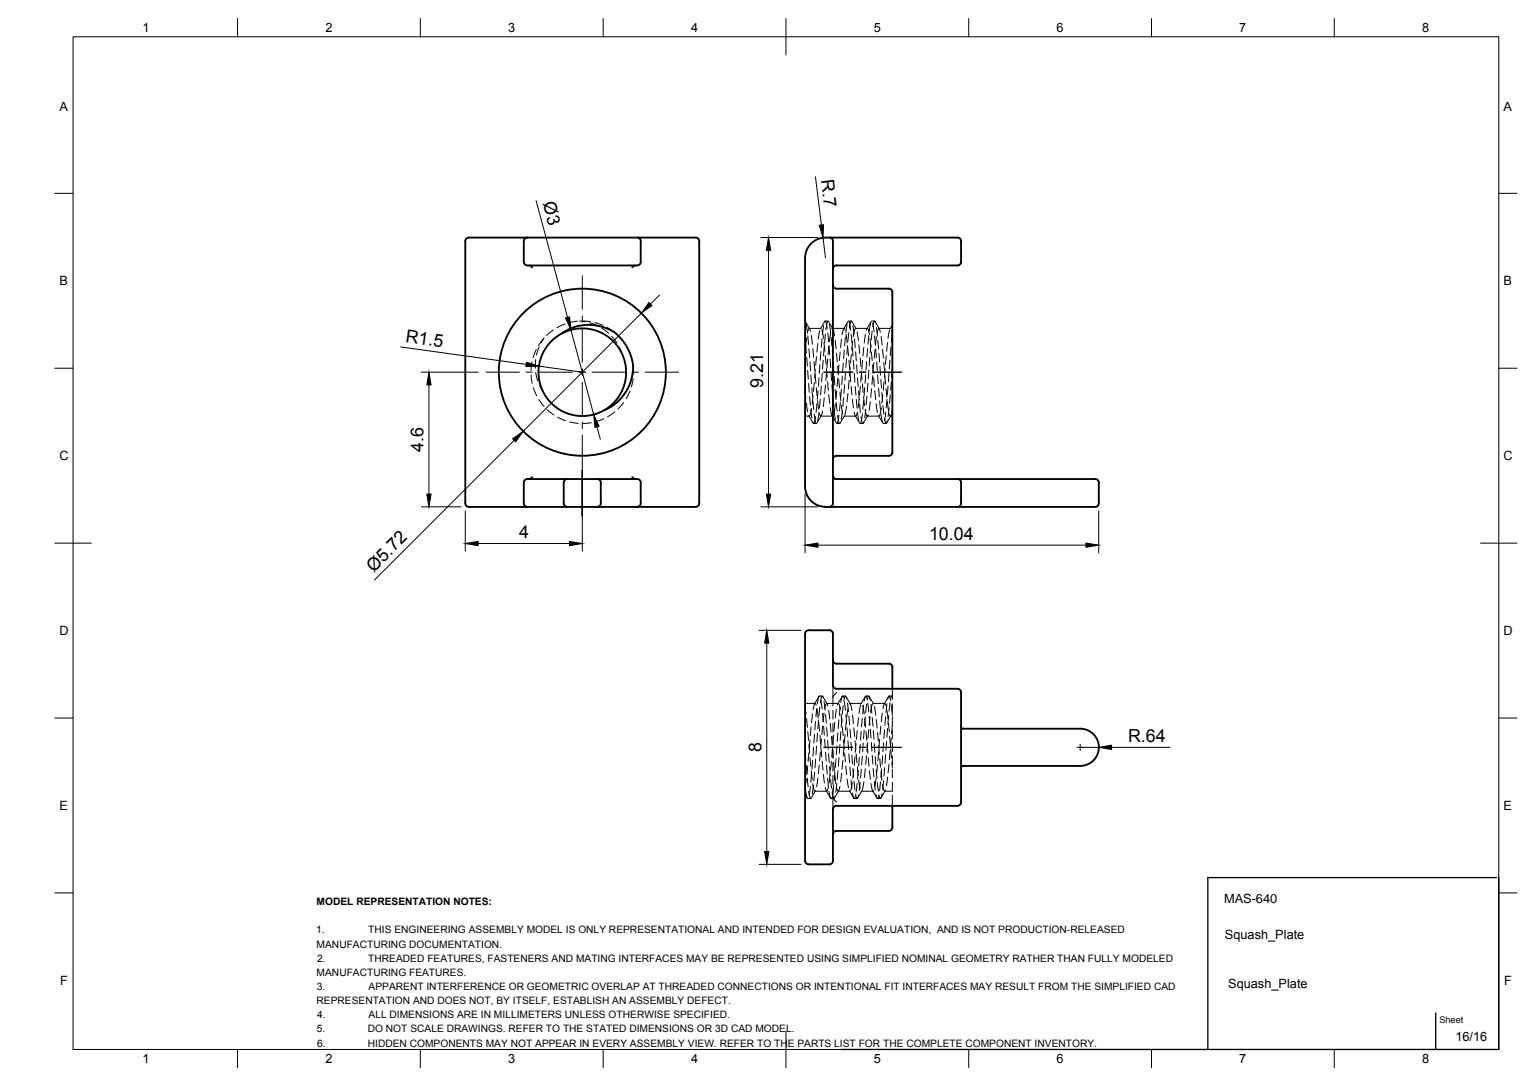
ISO-10303-21;
HEADER;
FILE_DESCRIPTION((''),'2;1');
FILE_NAME('Squash_Plate.step','2026-10-09T10:33:02-07:00',(''),(''),'','','');
FILE_SCHEMA (('AUTOMOTIVE_DESIGN { 1 0 10303 214 3 1 1 }'));
ENDSEC;
DATA;
#10=MECHANICAL_DESIGN_GEOMETRIC_PRESENTATION_REPRESENTATION('',(#844),#86330);
#109=SPHERICAL_SURFACE('',#35974,0.125) ;
#110=SPHERICAL_SURFACE('',#35976,0.125) ;
#111=SPHERICAL_SURFACE('',#35981,0.125) ;
#112=SPHERICAL_SURFACE('',#35983,0.125) ;
#113=SPHERICAL_SURFACE('',#36041,0.125) ;
#114=SPHERICAL_SURFACE('',#36047,0.125) ;
#115=SPHERICAL_SURFACE('',#36104,0.124999999999993) ;
#116=SPHERICAL_SURFACE('',#36105,0.125000000000011) ;
#117=SPHERICAL_SURFACE('',#36116,0.124999999999993) ;
#118=SPHERICAL_SURFACE('',#36117,0.124999999999993) ;
#119=SPHERICAL_SURFACE('',#36118,0.124999999999993) ;
#120=SPHERICAL_SURFACE('',#36119,0.124999999999993) ;
#436=TOROIDAL_SURFACE('',#35930,0.188499999999969,0.124999999999993) ;
#437=TOROIDAL_SURFACE('',#35937,0.188499999999987,0.124999999999993) ;
#438=TOROIDAL_SURFACE('',#35942,0.188499999999987,0.124999999999993) ;
#439=TOROIDAL_SURFACE('',#35949,0.509999999999996,0.125) ;
#440=TOROIDAL_SURFACE('',#35956,0.188499999999987,0.124999999999993) ;
#441=TOROIDAL_SURFACE('',#35965,0.509999999999996,0.125) ;
#442=TOROIDAL_SURFACE('',#36032,0.25,0.125) ;
#443=TOROIDAL_SURFACE('',#36035,0.25,0.125) ;
#444=TOROIDAL_SURFACE('',#36038,0.25,0.125) ;
#445=TOROIDAL_SURFACE('',#36044,0.25,0.125) ;
#446=TOROIDAL_SURFACE('',#36064,0.573499999999999,0.125) ;
#447=TOROIDAL_SURFACE('',#36068,0.573500000000001,0.125) ;
#448=TOROIDAL_SURFACE('',#36081,0.573500000000001,0.125) ;
#449=TOROIDAL_SURFACE('',#36085,0.573499999999999,0.125) ;
#450=TOROIDAL_SURFACE('',#36111,0.249999999999986,0.124999999999993) ;
#451=TOROIDAL_SURFACE('',#36115,0.250000000000004,0.124999999999993) ;
#452=TOROIDAL_SURFACE('',#36120,0.249999999999968,0.124999999999993) ;
#453=TOROIDAL_SURFACE('',#36121,0.249999999999986,0.124999999999993) ;
#454=TOROIDAL_SURFACE('',#36122,2.7325,0.125) ;
#455=TOROIDAL_SURFACE('',#36131,2.9825,0.125) ;
#746=(
BOUNDED_SURFACE()
B_SPLINE_SURFACE(1,2,((#79923,#79924,#79925,#79926,#79927,#79928,#79929,
#79930,#79931,#79932,#79933,#79934,#79935,#79936,#79937,#79938,#79939,#79940,
#79941,#79942,#79943,#79944,#79945,#79946,#79947,#79948,#79949,#79950,#79951,
#79952,#79953,#79954,#79955,#79956,#79957,#79958,#79959,#79960,#79961,#79962,
#79963,#79964,#79965,#79966,#79967,#79968,#79969,#79970,#79971,#79972,#79973,
#79974,#79975,#79976,#79977,#79978,#79979,#79980,#79981,#79982,#79983,#79984,
#79985,#79986,#79987,#79988,#79989,#79990,#79991,#79992,#79993,#79994,#79995,
#79996,#79997,#79998,#79999,#80000,#80001,#80002,#80003,#80004,#80005,#80006,
#80007,#80008,#80009,#80010,#80011,#80012,#80013,#80014,#80015,#80016,#80017,
#80018,#80019,#80020,#80021,#80022,#80023,#80024,#80025,#80026,#80027,#80028,
#80029,#80030,#80031,#80032,#80033,#80034,#80035,#80036,#80037,#80038,#80039,
#80040,#80041,#80042,#80043,#80044,#80045,#80046,#80047,#80048,#80049,#80050,
#80051,#80052,#80053,#80054,#80055,#80056,#80057,#80058,#80059,#80060,#80061,
#80062,#80063,#80064,#80065,#80066,#80067),(#80068,#80069,#80070,#80071,
#80072,#80073,#80074,#80075,#80076,#80077,#80078,#80079,#80080,#80081,#80082,
#80083,#80084,#80085,#80086,#80087,#80088,#80089,#80090,#80091,#80092,#80093,
#80094,#80095,#80096,#80097,#80098,#80099,#80100,#80101,#80102,#80103,#80104,
#80105,#80106,#80107,#80108,#80109,#80110,#80111,#80112,#80113,#80114,#80115,
#80116,#80117,#80118,#80119,#80120,#80121,#80122,#80123,#80124,#80125,#80126,
#80127,#80128,#80129,#80130,#80131,#80132,#80133,#80134,#80135,#80136,#80137,
#80138,#80139,#80140,#80141,#80142,#80143,#80144,#80145,#80146,#80147,#80148,
#80149,#80150,#80151,#80152,#80153,#80154,#80155,#80156,#80157,#80158,#80159,
#80160,#80161,#80162,#80163,#80164,#80165,#80166,#80167,#80168,#80169,#80170,
#80171,#80172,#80173,#80174,#80175,#80176,#80177,#80178,#80179,#80180,#80181,
#80182,#80183,#80184,#80185,#80186,#80187,#80188,#80189,#80190,#80191,#80192,
#80193,#80194,#80195,#80196,#80197,#80198,#80199,#80200,#80201,#80202,#80203,
#80204,#80205,#80206,#80207,#80208,#80209,#80210,#80211,#80212),(#80213,
#80214,#80215,#80216,#80217,#80218,#80219,#80220,#80221,#80222,#80223,#80224,
#80225,#80226,#80227,#80228,#80229,#80230,#80231,#80232,#80233,#80234,#80235,
#80236,#80237,#80238,#80239,#80240,#80241,#80242,#80243,#80244,#80245,#80246,
#80247,#80248,#80249,#80250,#80251,#80252,#80253,#80254,#80255,#80256,#80257,
#80258,#80259,#80260,#80261,#80262,#80263,#80264,#80265,#80266,#80267,#80268,
#80269,#80270,#80271,#80272,#80273,#80274,#80275,#80276,#80277,#80278,#80279,
#80280,#80281,#80282,#80283,#80284,#80285,#80286,#80287,#80288,#80289,#80290,
#80291,#80292,#80293,#80294,#80295,#80296,#80297,#80298,#80299,#80300,#80301,
#80302,#80303,#80304,#80305,#80306,#80307,#80308,#80309,#80310,#80311,#80312,
#80313,#80314,#80315,#80316,#80317,#80318,#80319,#80320,#80321,#80322,#80323,
#80324,#80325,#80326,#80327,#80328,#80329,#80330,#80331,#80332,#80333,#80334,
#80335,#80336,#80337,#80338,#80339,#80340,#80341,#80342,#80343,#80344,#80345,
#80346,#80347,#80348,#80349,#80350,#80351,#80352,#80353,#80354,#80355,#80356,
#80357),(#80358,#80359,#80360,#80361,#80362,#80363,#80364,#80365,#80366,
#80367,#80368,#80369,#80370,#80371,#80372,#80373,#80374,#80375,#80376,#80377,
#80378,#80379,#80380,#80381,#80382,#80383,#80384,#80385,#80386,#80387,#80388,
#80389,#80390,#80391,#80392,#80393,#80394,#80395,#80396,#80397,#80398,#80399,
#80400,#80401,#80402,#80403,#80404,#80405,#80406,#80407,#80408,#80409,#80410,
#80411,#80412,#80413,#80414,#80415,#80416,#80417,#80418,#80419,#80420,#80421,
#80422,#80423,#80424,#80425,#80426,#80427,#80428,#80429,#80430,#80431,#80432,
#80433,#80434,#80435,#80436,#80437,#80438,#80439,#80440,#80441,#80442,#80443,
#80444,#80445,#80446,#80447,#80448,#80449,#80450,#80451,#80452,#80453,#80454,
#80455,#80456,#80457,#80458,#80459,#80460,#80461,#80462,#80463,#80464,#80465,
#80466,#80467,#80468,#80469,#80470,#80471,#80472,#80473,#80474,#80475,#80476,
#80477,#80478,#80479,#80480,#80481,#80482,#80483,#80484,#80485,#80486,#80487,
#80488,#80489,#80490,#80491,#80492,#80493,#80494,#80495,#80496,#80497,#80498,
#80499,#80500,#80501,#80502)),.UNSPECIFIED.,.F.,.F.,.F.)
B_SPLINE_SURFACE_WITH_KNOTS((2,1,1,2),(3,2,2,2,2,2,2,2,2,2,2,2,2,2,2,2,
2,2,2,2,2,2,2,2,2,2,2,2,2,2,2,2,2,2,2,2,2,2,2,2,2,2,2,2,2,2,2,2,2,2,2,2,
2,2,2,2,2,2,2,2,2,2,2,2,2,2,2,2,2,2,2,2,3),(-5.32860868657006,0.,1.,2.58924025826637),
(0.,0.0138888888888889,0.0277777777777778,0.0416666666666667,0.0555555555555556,
0.0694444444444444,0.0833333333333333,0.0972222222222222,0.111111111111111,
0.125,0.138888888888889,0.152777777777778,0.166666666666667,0.180555555555556,
0.194444444444444,0.208333333333333,0.222222222222222,0.236111111111111,
0.25,0.263888888888889,0.277777777777778,0.291666666666667,0.305555555555556,
0.319444444444444,0.333333333333333,0.347222222222222,0.361111111111111,
0.375,0.388888888888889,0.402777777777778,0.416666666666667,0.430555555555556,
0.444444444444444,0.458333333333333,0.472222222222222,0.486111111111111,
0.5,0.513888888888889,0.527777777777778,0.541666666666667,0.555555555555556,
0.569444444444444,0.583333333333333,0.597222222222222,0.611111111111111,
0.625,0.638888888888889,0.652777777777778,0.666666666666667,0.680555555555556,
0.694444444444444,0.708333333333333,0.722222222222222,0.736111111111111,
0.75,0.763888888888889,0.777777777777778,0.791666666666667,0.805555555555556,
0.819444444444444,0.833333333333333,0.847222222222222,0.861111111111111,
0.875,0.888888888888889,0.902777777777778,0.916666666666667,0.930555555555556,
0.944444444444444,0.958333333333333,0.972222222222222,0.986111111111111,
1.),.UNSPECIFIED.)
GEOMETRIC_REPRESENTATION_ITEM()
RATIONAL_B_SPLINE_SURFACE(((1.,0.923879532511287,1.,0.923879532511287,1.,
0.923879532511287,1.,0.923879532511287,1.,0.923879532511287,1.,0.923879532511287,
1.,0.923879532511287,1.,0.923879532511287,1.,0.923879532511287,1.,0.923879532511287,
1.,0.923879532511287,1.,0.923879532511287,1.,0.923879532511287,1.,0.923879532511287,
1.,0.923879532511287,1.,0.923879532511287,1.,0.923879532511287,1.,0.923879532511287,
1.,0.923879532511287,1.,0.923879532511287,1.,0.923879532511287,1.,0.923879532511287,
1.,0.923879532511287,1.,0.923879532511287,1.,0.923879532511287,1.,0.923879532511287,
1.,0.923879532511287,1.,0.923879532511287,1.,0.923879532511287,1.,0.923879532511287,
1.,0.923879532511287,1.,0.923879532511287,1.,0.923879532511287,1.,0.923879532511287,
1.,0.923879532511287,1.,0.923879532511287,1.,0.923879532511287,1.,0.923879532511287,
1.,0.923879532511287,1.,0.923879532511287,1.,0.923879532511287,1.,0.923879532511287,
1.,0.923879532511287,1.,0.923879532511287,1.,0.923879532511287,1.,0.923879532511287,
1.,0.923879532511287,1.,0.923879532511287,1.,0.923879532511287,1.,0.923879532511287,
1.,0.923879532511287,1.,0.923879532511287,1.,0.923879532511287,1.,0.923879532511287,
1.,0.923879532511287,1.,0.923879532511287,1.,0.923879532511287,1.,0.923879532511287,
1.,0.923879532511287,1.,0.923879532511287,1.,0.923879532511287,1.,0.923879532511287,
1.,0.923879532511287,1.,0.923879532511287,1.,0.923879532511287,1.,0.923879532511287,
1.,0.923879532511287,1.,0.923879532511287,1.,0.923879532511287,1.,0.923879532511287,
1.,0.923879532511287,1.,0.923879532511287,1.),(1.,0.923879532511287,1.,
0.923879532511287,1.,0.923879532511287,1.,0.923879532511287,1.,0.923879532511287,
1.,0.923879532511287,1.,0.923879532511287,1.,0.923879532511287,1.,0.923879532511287,
1.,0.923879532511287,1.,0.923879532511287,1.,0.923879532511287,1.,0.923879532511287,
1.,0.923879532511287,1.,0.923879532511287,1.,0.923879532511287,1.,0.923879532511287,
1.,0.923879532511287,1.,0.923879532511287,1.,0.923879532511287,1.,0.923879532511287,
1.,0.923879532511287,1.,0.923879532511287,1.,0.923879532511287,1.,0.923879532511287,
1.,0.923879532511287,1.,0.923879532511287,1.,0.923879532511287,1.,0.923879532511287,
1.,0.923879532511287,1.,0.923879532511287,1.,0.923879532511287,1.,0.923879532511287,
1.,0.923879532511287,1.,0.923879532511287,1.,0.923879532511287,1.,0.923879532511287,
1.,0.923879532511287,1.,0.923879532511287,1.,0.923879532511287,1.,0.923879532511287,
1.,0.923879532511287,1.,0.923879532511287,1.,0.923879532511287,1.,0.923879532511287,
1.,0.923879532511287,1.,0.923879532511287,1.,0.923879532511287,1.,0.923879532511287,
1.,0.923879532511287,1.,0.923879532511287,1.,0.923879532511287,1.,0.923879532511287,
1.,0.923879532511287,1.,0.923879532511287,1.,0.923879532511287,1.,0.923879532511287,
1.,0.923879532511287,1.,0.923879532511287,1.,0.923879532511287,1.,0.923879532511287,
1.,0.923879532511287,1.,0.923879532511287,1.,0.923879532511287,1.,0.923879532511287,
1.,0.923879532511287,1.,0.923879532511287,1.,0.923879532511287,1.,0.923879532511287,
1.,0.923879532511287,1.,0.923879532511287,1.,0.923879532511287,1.),(1.,
0.923879532511287,1.,0.923879532511287,1.,0.923879532511287,1.,0.923879532511287,
1.,0.923879532511287,1.,0.923879532511287,1.,0.923879532511287,1.,0.923879532511287,
1.,0.923879532511287,1.,0.923879532511287,1.,0.923879532511287,1.,0.923879532511287,
1.,0.923879532511287,1.,0.923879532511287,1.,0.923879532511287,1.,0.923879532511287,
1.,0.923879532511287,1.,0.923879532511287,1.,0.923879532511287,1.,0.923879532511287,
1.,0.923879532511287,1.,0.923879532511287,1.,0.923879532511287,1.,0.923879532511287,
1.,0.923879532511287,1.,0.923879532511287,1.,0.923879532511287,1.,0.923879532511287,
1.,0.923879532511287,1.,0.923879532511287,1.,0.923879532511287,1.,0.923879532511287,
1.,0.923879532511287,1.,0.923879532511287,1.,0.923879532511287,1.,0.923879532511287,
1.,0.923879532511287,1.,0.923879532511287,1.,0.923879532511287,1.,0.923879532511287,
1.,0.923879532511287,1.,0.923879532511287,1.,0.923879532511287,1.,0.923879532511287,
1.,0.923879532511287,1.,0.923879532511287,1.,0.923879532511287,1.,0.923879532511287,
1.,0.923879532511287,1.,0.923879532511287,1.,0.923879532511287,1.,0.923879532511287,
1.,0.923879532511287,1.,0.923879532511287,1.,0.923879532511287,1.,0.923879532511287,
1.,0.923879532511287,1.,0.923879532511287,1.,0.923879532511287,1.,0.923879532511287,
1.,0.923879532511287,1.,0.923879532511287,1.,0.923879532511287,1.,0.923879532511287,
1.,0.923879532511287,1.,0.923879532511287,1.,0.923879532511287,1.,0.923879532511287,
1.,0.923879532511287,1.,0.923879532511287,1.,0.923879532511287,1.,0.923879532511287,
1.),(1.,0.923879532511287,1.,0.923879532511287,1.,0.923879532511287,1.,
0.923879532511287,1.,0.923879532511287,1.,0.923879532511287,1.,0.923879532511287,
1.,0.923879532511287,1.,0.923879532511287,1.,0.923879532511287,1.,0.923879532511287,
1.,0.923879532511287,1.,0.923879532511287,1.,0.923879532511287,1.,0.923879532511287,
1.,0.923879532511287,1.,0.923879532511287,1.,0.923879532511287,1.,0.923879532511287,
1.,0.923879532511287,1.,0.923879532511287,1.,0.923879532511287,1.,0.923879532511287,
1.,0.923879532511287,1.,0.923879532511287,1.,0.923879532511287,1.,0.923879532511287,
1.,0.923879532511287,1.,0.923879532511287,1.,0.923879532511287,1.,0.923879532511287,
1.,0.923879532511287,1.,0.923879532511287,1.,0.923879532511287,1.,0.923879532511287,
1.,0.923879532511287,1.,0.923879532511287,1.,0.923879532511287,1.,0.923879532511287,
1.,0.923879532511287,1.,0.923879532511287,1.,0.923879532511287,1.,0.923879532511287,
1.,0.923879532511287,1.,0.923879532511287,1.,0.923879532511287,1.,0.923879532511287,
1.,0.923879532511287,1.,0.923879532511287,1.,0.923879532511287,1.,0.923879532511287,
1.,0.923879532511287,1.,0.923879532511287,1.,0.923879532511287,1.,0.923879532511287,
1.,0.923879532511287,1.,0.923879532511287,1.,0.923879532511287,1.,0.923879532511287,
1.,0.923879532511287,1.,0.923879532511287,1.,0.923879532511287,1.,0.923879532511287,
1.,0.923879532511287,1.,0.923879532511287,1.,0.923879532511287,1.,0.923879532511287,
1.,0.923879532511287,1.,0.923879532511287,1.,0.923879532511287,1.,0.923879532511287,
1.,0.923879532511287,1.)))
REPRESENTATION_ITEM('')
SURFACE()
) ;
#747=(
BOUNDED_SURFACE()
B_SPLINE_SURFACE(1,2,((#80503,#80504,#80505,#80506,#80507,#80508,#80509,
#80510,#80511,#80512,#80513,#80514,#80515,#80516,#80517,#80518,#80519,#80520,
#80521,#80522,#80523,#80524,#80525,#80526,#80527,#80528,#80529,#80530,#80531,
#80532,#80533,#80534,#80535,#80536,#80537,#80538,#80539,#80540,#80541,#80542,
#80543,#80544,#80545,#80546,#80547,#80548,#80549,#80550,#80551,#80552,#80553,
#80554,#80555,#80556,#80557,#80558,#80559,#80560,#80561,#80562,#80563,#80564,
#80565,#80566,#80567,#80568,#80569,#80570,#80571,#80572,#80573,#80574,#80575,
#80576,#80577,#80578,#80579,#80580,#80581,#80582,#80583,#80584,#80585,#80586,
#80587,#80588,#80589,#80590,#80591,#80592,#80593,#80594,#80595,#80596,#80597,
#80598,#80599,#80600,#80601,#80602,#80603,#80604,#80605,#80606,#80607,#80608,
#80609,#80610,#80611,#80612,#80613,#80614,#80615,#80616,#80617,#80618,#80619,
#80620,#80621,#80622,#80623,#80624,#80625,#80626,#80627,#80628,#80629,#80630,
#80631,#80632,#80633,#80634,#80635,#80636,#80637,#80638,#80639,#80640,#80641,
#80642,#80643,#80644,#80645,#80646,#80647),(#80648,#80649,#80650,#80651,
#80652,#80653,#80654,#80655,#80656,#80657,#80658,#80659,#80660,#80661,#80662,
#80663,#80664,#80665,#80666,#80667,#80668,#80669,#80670,#80671,#80672,#80673,
#80674,#80675,#80676,#80677,#80678,#80679,#80680,#80681,#80682,#80683,#80684,
#80685,#80686,#80687,#80688,#80689,#80690,#80691,#80692,#80693,#80694,#80695,
#80696,#80697,#80698,#80699,#80700,#80701,#80702,#80703,#80704,#80705,#80706,
#80707,#80708,#80709,#80710,#80711,#80712,#80713,#80714,#80715,#80716,#80717,
#80718,#80719,#80720,#80721,#80722,#80723,#80724,#80725,#80726,#80727,#80728,
#80729,#80730,#80731,#80732,#80733,#80734,#80735,#80736,#80737,#80738,#80739,
#80740,#80741,#80742,#80743,#80744,#80745,#80746,#80747,#80748,#80749,#80750,
#80751,#80752,#80753,#80754,#80755,#80756,#80757,#80758,#80759,#80760,#80761,
#80762,#80763,#80764,#80765,#80766,#80767,#80768,#80769,#80770,#80771,#80772,
#80773,#80774,#80775,#80776,#80777,#80778,#80779,#80780,#80781,#80782,#80783,
#80784,#80785,#80786,#80787,#80788,#80789,#80790,#80791,#80792)),
 .UNSPECIFIED.,.F.,.F.,.F.)
B_SPLINE_SURFACE_WITH_KNOTS((2,2),(3,2,2,2,2,2,2,2,2,2,2,2,2,2,2,2,2,2,
2,2,2,2,2,2,2,2,2,2,2,2,2,2,2,2,2,2,2,2,2,2,2,2,2,2,2,2,2,2,2,2,2,2,2,2,
2,2,2,2,2,2,2,2,2,2,2,2,2,2,2,2,2,2,3),(0.,1.00004424589271),(0.,0.0138888888888889,
0.0277777777777778,0.0416666666666667,0.0555555555555556,0.0694444444444444,
0.0833333333333333,0.0972222222222222,0.111111111111111,0.125,0.138888888888889,
0.152777777777778,0.166666666666667,0.180555555555556,0.194444444444444,
0.208333333333333,0.222222222222222,0.236111111111111,0.25,0.263888888888889,
0.277777777777778,0.291666666666667,0.305555555555556,0.319444444444444,
0.333333333333333,0.347222222222222,0.361111111111111,0.375,0.388888888888889,
0.402777777777778,0.416666666666667,0.430555555555556,0.444444444444444,
0.458333333333333,0.472222222222222,0.486111111111111,0.5,0.513888888888889,
0.527777777777778,0.541666666666667,0.555555555555556,0.569444444444444,
0.583333333333333,0.597222222222222,0.611111111111111,0.625,0.638888888888889,
0.652777777777778,0.666666666666667,0.680555555555556,0.694444444444444,
0.708333333333333,0.722222222222222,0.736111111111111,0.75,0.763888888888889,
0.777777777777778,0.791666666666667,0.805555555555556,0.819444444444444,
0.833333333333333,0.847222222222222,0.861111111111111,0.875,0.888888888888889,
0.902777777777778,0.916666666666667,0.930555555555556,0.944444444444444,
0.958333333333333,0.972222222222222,0.986111111111111,1.),.UNSPECIFIED.)
GEOMETRIC_REPRESENTATION_ITEM()
RATIONAL_B_SPLINE_SURFACE(((1.,0.923879532511287,1.,0.923879532511287,1.,
0.923879532511287,1.,0.923879532511287,1.,0.923879532511287,1.,0.923879532511287,
1.,0.923879532511287,1.,0.923879532511287,1.,0.923879532511287,1.,0.923879532511287,
1.,0.923879532511287,1.,0.923879532511287,1.,0.923879532511287,1.,0.923879532511287,
1.,0.923879532511287,1.,0.923879532511287,1.,0.923879532511287,1.,0.923879532511287,
1.,0.923879532511287,1.,0.923879532511287,1.,0.923879532511287,1.,0.923879532511287,
1.,0.923879532511287,1.,0.923879532511287,1.,0.923879532511287,1.,0.923879532511287,
1.,0.923879532511287,1.,0.923879532511287,1.,0.923879532511287,1.,0.923879532511287,
1.,0.923879532511287,1.,0.923879532511287,1.,0.923879532511287,1.,0.923879532511287,
1.,0.923879532511287,1.,0.923879532511287,1.,0.923879532511287,1.,0.923879532511287,
1.,0.923879532511287,1.,0.923879532511287,1.,0.923879532511287,1.,0.923879532511287,
1.,0.923879532511287,1.,0.923879532511287,1.,0.923879532511287,1.,0.923879532511287,
1.,0.923879532511287,1.,0.923879532511287,1.,0.923879532511287,1.,0.923879532511287,
1.,0.923879532511287,1.,0.923879532511287,1.,0.923879532511287,1.,0.923879532511287,
1.,0.923879532511287,1.,0.923879532511287,1.,0.923879532511287,1.,0.923879532511287,
1.,0.923879532511287,1.,0.923879532511287,1.,0.923879532511287,1.,0.923879532511287,
1.,0.923879532511287,1.,0.923879532511287,1.,0.923879532511287,1.,0.923879532511287,
1.,0.923879532511287,1.,0.923879532511287,1.,0.923879532511287,1.,0.923879532511287,
1.,0.923879532511287,1.,0.923879532511287,1.),(1.,0.923879532511287,1.,
0.923879532511287,1.,0.923879532511287,1.,0.923879532511287,1.,0.923879532511287,
1.,0.923879532511287,1.,0.923879532511287,1.,0.923879532511287,1.,0.923879532511287,
1.,0.923879532511287,1.,0.923879532511287,1.,0.923879532511287,1.,0.923879532511287,
1.,0.923879532511287,1.,0.923879532511287,1.,0.923879532511287,1.,0.923879532511287,
1.,0.923879532511287,1.,0.923879532511287,1.,0.923879532511287,1.,0.923879532511287,
1.,0.923879532511287,1.,0.923879532511287,1.,0.923879532511287,1.,0.923879532511287,
1.,0.923879532511287,1.,0.923879532511287,1.,0.923879532511287,1.,0.923879532511287,
1.,0.923879532511287,1.,0.923879532511287,1.,0.923879532511287,1.,0.923879532511287,
1.,0.923879532511287,1.,0.923879532511287,1.,0.923879532511287,1.,0.923879532511287,
1.,0.923879532511287,1.,0.923879532511287,1.,0.923879532511287,1.,0.923879532511287,
1.,0.923879532511287,1.,0.923879532511287,1.,0.923879532511287,1.,0.923879532511287,
1.,0.923879532511287,1.,0.923879532511287,1.,0.923879532511287,1.,0.923879532511287,
1.,0.923879532511287,1.,0.923879532511287,1.,0.923879532511287,1.,0.923879532511287,
1.,0.923879532511287,1.,0.923879532511287,1.,0.923879532511287,1.,0.923879532511287,
1.,0.923879532511287,1.,0.923879532511287,1.,0.923879532511287,1.,0.923879532511287,
1.,0.923879532511287,1.,0.923879532511287,1.,0.923879532511287,1.,0.923879532511287,
1.,0.923879532511287,1.,0.923879532511287,1.,0.923879532511287,1.,0.923879532511287,
1.,0.923879532511287,1.,0.923879532511287,1.,0.923879532511287,1.)))
REPRESENTATION_ITEM('')
SURFACE()
) ;
#820=SHAPE_REPRESENTATION_RELATIONSHIP('SRR','None',#86465,#832) ;
#832=ADVANCED_BREP_SHAPE_REPRESENTATION('',(#856),#86319) ;
#844=STYLED_ITEM('',(#86582),#856) ;
#856=MANIFOLD_SOLID_BREP('Body1',#32643) ;
#1170=FACE_BOUND('',#5960,.T.) ;
#1171=FACE_BOUND('',#6015,.T.) ;
#1172=FACE_BOUND('',#6019,.T.) ;
#1580=B_SPLINE_CURVE_WITH_KNOTS('',3,(#78793,#78794,#78795,#78796,#78797,
#78798,#78799,#78800,#78801,#78802,#78803,#78804,#78805,#78806,#78807,#78808),
 .UNSPECIFIED.,.F.,.F.,(4,2,2,2,2,2,2,4),(3.73678905355268,3.77583604564174,
3.84429316886454,3.9117839455625,3.98028517515954,4.04771812918815,4.09356285357691,
4.13893020482044),.UNSPECIFIED.) ;
#1581=B_SPLINE_CURVE_WITH_KNOTS('',3,(#78811,#78812,#78813,#78814,#78815,
#78816,#78817,#78818,#78819,#78820,#78821,#78822,#78823,#78824,#78825,#78826,
#78827,#78828,#78829,#78830),.UNSPECIFIED.,.F.,.F.,(4,2,2,2,2,2,2,2,2,4),
(1.00000010744283E-6,0.0499431784479235,0.100287210935025,0.168054642610065,
0.237494946806667,0.305292985567466,0.374683046548786,0.442516172111994,
0.51185655028286,0.544247303702404),.UNSPECIFIED.) ;
#1582=B_SPLINE_CURVE_WITH_KNOTS('',3,(#78835,#78836,#78837,#78838,#78839,
#78840,#78841,#78842,#78843,#78844,#78845,#78846,#78847,#78848,#78849,#78850,
#78851,#78852,#78853,#78854,#78855,#78856,#78857,#78858,#78859,#78860,#78861,
#78862,#78863,#78864,#78865,#78866,#78867,#78868,#78869,#78870),
 .UNSPECIFIED.,.F.,.F.,(4,2,2,2,2,2,2,2,2,2,2,2,2,2,2,2,2,4),(2.63879249403916,
2.68716207519284,2.75533111613759,2.82339735412774,2.89159459627009,2.95958001185233,
3.02780800755272,3.09571469311715,3.1639758471015,3.23180612291199,3.30010268233795,
3.36785909776552,3.43619314464488,3.50387847678256,3.57225192300491,3.63986917252862,
3.70828375765117,3.73678905355268),.UNSPECIFIED.) ;
#1583=B_SPLINE_CURVE_WITH_KNOTS('',3,(#78871,#78872,#78873,#78874,#78875,
#78876,#78877,#78878,#78879,#78880,#78881,#78882,#78883,#78884,#78885,#78886,
#78887,#78888,#78889,#78890,#78891,#78892,#78893,#78894,#78895,#78896,#78897,
#78898,#78899,#78900,#78901,#78902,#78903,#78904,#78905,#78906),
 .UNSPECIFIED.,.F.,.F.,(4,2,2,2,2,2,2,2,2,2,2,2,2,2,2,2,2,4),(0.544247303702404,
0.579729241383105,0.649020714981666,0.71693728891309,0.786180492040209,
0.854145311540051,0.923341134445988,0.991358342360499,1.06050780118652,
1.12858131963186,1.19768557917167,1.26581915872125,1.33487954264344,1.40307674572091,
1.47209474432328,1.54035893111266,1.6093362063892,1.65177826841052),
 .UNSPECIFIED.) ;
#1584=B_SPLINE_CURVE_WITH_KNOTS('',3,(#78911,#78912,#78913,#78914,#78915,
#78916,#78917,#78918,#78919,#78920,#78921,#78922,#78923,#78924,#78925,#78926,
#78927,#78928,#78929,#78930,#78931,#78932,#78933,#78934,#78935,#78936,#78937,
#78938,#78939,#78940,#78941,#78942,#78943,#78944,#78945,#78946),
 .UNSPECIFIED.,.F.,.F.,(4,2,2,2,2,2,2,2,2,2,2,2,2,2,2,2,2,4),(1.5389994522091,
1.59333149801295,1.66297884651135,1.7301821776633,1.79977280875785,1.86694772145314,
1.93648225696496,2.00363195036966,2.07311098033212,2.14160511265088,2.20968937196864,
2.27809543856464,2.34619647664059,2.41451552535451,2.48263634985671,2.55086961886095,
2.61901314661333,2.63879249403916),.UNSPECIFIED.) ;
#1585=B_SPLINE_CURVE_WITH_KNOTS('',3,(#78947,#78948,#78949,#78950,#78951,
#78952,#78953,#78954,#78955,#78956,#78957,#78958,#78959,#78960,#78961,#78962,
#78963,#78964,#78965,#78966,#78967,#78968,#78969,#78970,#78971,#78972,#78973,
#78974,#78975,#78976,#78977,#78978,#78979,#78980,#78981,#78982),
 .UNSPECIFIED.,.F.,.F.,(4,2,2,2,2,2,2,2,2,2,2,2,2,2,2,2,2,4),(1.65177826841052,
1.6776705234471,1.7466089112996,1.81501628298846,1.8839177925435,1.95240091532547,
2.02126772540027,2.08982906495714,2.15959253692843,2.22727314697463,2.29708965878139,
2.36477169799653,2.43464163209697,2.50232925343889,2.57225301932284,2.63995025192664,
2.70992829083685,2.76015985424245),.UNSPECIFIED.) ;
#1586=B_SPLINE_CURVE_WITH_KNOTS('',3,(#78988,#78989,#78990,#78991,#78992,
#78993,#78994,#78995,#78996,#78997,#78998,#78999,#79000,#79001),
 .UNSPECIFIED.,.F.,.F.,(4,2,2,2,2,2,4),(3.87088446641146,3.88207110309913,
3.95256288258768,4.02054495054698,4.09109719843181,4.13081697342442,4.16975042780213),
 .UNSPECIFIED.) ;
#1587=B_SPLINE_CURVE_WITH_KNOTS('',3,(#79004,#79005,#79006,#79007,#79008,
#79009,#79010,#79011,#79012,#79013,#79014,#79015,#79016,#79017,#79018,#79019,
#79020,#79021),.UNSPECIFIED.,.F.,.F.,(4,2,2,2,2,2,2,2,4),(9.99925951688718E-7,
0.0402770593329322,0.0813965593939245,0.151714020497245,0.219397414529146,
0.289650306659335,0.357279908909674,0.427468950574574,0.435597230048873),
 .UNSPECIFIED.) ;
#1588=B_SPLINE_CURVE_WITH_KNOTS('',3,(#79027,#79028,#79029,#79030,#79031,
#79032,#79033,#79034,#79035,#79036),.UNSPECIFIED.,.F.,.F.,(4,2,2,2,4),(-0.1667127750087,
-0.142097710392982,-0.0825624075964315,-0.0415013685793908,-1.00000012634438E-6),
 .UNSPECIFIED.) ;
#1589=B_SPLINE_CURVE_WITH_KNOTS('',3,(#79039,#79040,#79041,#79042,#79043,
#79044,#79045,#79046,#79047,#79048,#79049,#79050,#79051,#79052,#79053,#79054,
#79055,#79056,#79057,#79058,#79059,#79060,#79061,#79062,#79063,#79064),
 .UNSPECIFIED.,.F.,.F.,(4,2,2,2,2,2,2,2,2,2,2,2,4),(-3.52511524228821,-3.4879111620666,
-3.45147286206197,-3.39356408207001,-3.33588355377615,-3.27799407259938,
-3.22024929076642,-3.16237686440599,-3.10456617477217,-3.04670845322558,
-2.98883032321556,-2.9309848603785,-2.88876551162052),.UNSPECIFIED.) ;
#1590=B_SPLINE_CURVE_WITH_KNOTS('',3,(#79069,#79070,#79071,#79072,#79073,
#79074,#79075,#79076,#79077,#79078,#79079,#79080,#79081,#79082,#79083,#79084,
#79085,#79086,#79087,#79088,#79089,#79090,#79091,#79092,#79093,#79094,#79095,
#79096,#79097,#79098,#79099,#79100,#79101,#79102,#79103,#79104),
 .UNSPECIFIED.,.F.,.F.,(4,2,2,2,2,2,2,2,2,2,2,2,2,2,2,2,2,4),(-1.1147036297923,
-1.08234127378787,-1.0231056786126,-0.964814237103067,-0.905544180711381,
-0.847294503532792,-0.787988947858243,-0.729777999922997,-0.670436005006492,
-0.612260463830717,-0.552881168011551,-0.494737717697047,-0.435320348351732,
-0.377205696945116,-0.317749544705521,-0.259660335123111,-0.200164740500403,
-0.1667127750087),.UNSPECIFIED.) ;
#1591=B_SPLINE_CURVE_WITH_KNOTS('',3,(#79105,#79106,#79107,#79108,#79109,
#79110,#79111,#79112,#79113,#79114,#79115,#79116,#79117,#79118,#79119,#79120,
#79121,#79122,#79123,#79124,#79125,#79126,#79127,#79128,#79129,#79130,#79131,
#79132,#79133,#79134,#79135,#79136,#79137,#79138,#79139,#79140),
 .UNSPECIFIED.,.F.,.F.,(4,2,2,2,2,2,2,2,2,2,2,2,2,2,2,2,2,4),(-2.88876551162052,
-2.8730378509001,-2.81520202632923,-2.75718479476445,-2.69935609300128,
-2.64126751092778,-2.58344326618254,-2.52528224276112,-2.46745974068091,
-2.40922528204208,-2.35140177232791,-2.2930929756667,-2.23526568453019,
-2.17688173210656,-2.1190478743858,-2.06058802751593,-2.00274481828321,
-1.95515401212426),.UNSPECIFIED.) ;
#1592=B_SPLINE_CURVE_WITH_KNOTS('',3,(#79145,#79146,#79147,#79148,#79149,
#79150,#79151,#79152,#79153,#79154,#79155,#79156,#79157,#79158,#79159,#79160,
#79161,#79162,#79163,#79164,#79165,#79166,#79167,#79168,#79169,#79170,#79171,
#79172,#79173,#79174,#79175,#79176,#79177,#79178,#79179,#79180),
 .UNSPECIFIED.,.F.,.F.,(4,2,2,2,2,2,2,2,2,2,2,2,2,2,2,2,2,4),(-2.06310075398818,
-2.02342933420803,-1.96363930695818,-1.90563613528142,-1.8458898927228,
-1.78788604802015,-1.72882872991433,-1.6702291728422,-1.61114617975511,
-1.5526042180681,-1.49349375729761,-1.43500706290225,-1.37586747600671,
-1.31743359143829,-1.25826335363796,-1.19987969503678,-1.1406774124604,
-1.1147036297923),.UNSPECIFIED.) ;
#1593=B_SPLINE_CURVE_WITH_KNOTS('',3,(#79181,#79182,#79183,#79184,#79185,
#79186,#79187,#79188,#79189,#79190,#79191,#79192,#79193,#79194,#79195,#79196,
#79197,#79198,#79199,#79200,#79201,#79202,#79203,#79204,#79205,#79206,#79207,
#79208,#79209,#79210,#79211,#79212,#79213,#79214,#79215,#79216),
 .UNSPECIFIED.,.F.,.F.,(4,2,2,2,2,2,2,2,2,2,2,2,2,2,2,2,2,4),(-1.95515401212426,
-1.94420841138501,-1.88635307691628,-1.82773951167999,-1.76986929968893,
-1.71260942538492,-1.65318316629389,-1.59587567208381,-1.53639019675408,
-1.47903330179993,-1.41948762790906,-1.36207963998264,-1.3024728018388,
-1.24501211437446,-1.18534316543117,-1.12782825442788,-1.06809626943629,
-1.01710396538768),.UNSPECIFIED.) ;
#1594=B_SPLINE_CURVE_WITH_KNOTS('',3,(#79222,#79223,#79224,#79225,#79226,
#79227,#79228,#79229),.UNSPECIFIED.,.F.,.F.,(4,2,2,4),(-0.0724080849059257,
-0.0675792623524678,-0.0340552227594196,-9.99999997836065E-7),
 .UNSPECIFIED.) ;
#1595=B_SPLINE_CURVE_WITH_KNOTS('',3,(#79232,#79233,#79234,#79235,#79236,
#79237,#79238,#79239,#79240,#79241,#79242,#79243,#79244,#79245,#79246,#79247,
#79248,#79249,#79250,#79251,#79252,#79253,#79254,#79255),.UNSPECIFIED.,
 .F.,.F.,(4,2,2,2,2,2,2,2,2,2,2,4),(-3.56932824666088,-3.53449866700443,
-3.50005253731909,-3.44177237096352,-3.38139391611913,-3.32315169324715,
-3.26282744772412,-3.2046207539918,-3.14434969751453,-3.08617601623974,
-3.02595714369959,-3.01323089524153),.UNSPECIFIED.) ;
#1596=B_SPLINE_CURVE_WITH_KNOTS('',3,(#79257,#79258,#79259,#79260,#79261,
#79262,#79263,#79264,#79265,#79266,#79267,#79268,#79269,#79270,#79271,#79272,
#79273,#79274,#79275,#79276,#79277,#79278,#79279,#79280,#79281,#79282,#79283,
#79284,#79285,#79286,#79287,#79288,#79289,#79290,#79291,#79292),
 .UNSPECIFIED.,.F.,.F.,(4,2,2,2,2,2,2,2,2,2,2,2,2,2,2,2,2,4),(-3.01323089524153,
-2.96781377424098,-2.90764599157684,-2.84953027391211,-2.78941272895961,
-2.73132186836034,-2.67125362853938,-2.61318471166392,-2.55316487653164,
-2.49511489832779,-2.43514260265038,-2.37710847123879,-2.31718288727562,
-2.2591614298491,-2.19928176867963,-2.14126973842676,-2.08143525016407,
-2.06310075398818),.UNSPECIFIED.) ;
#1597=B_SPLINE_CURVE_WITH_KNOTS('',3,(#79293,#79294,#79295,#79296,#79297,
#79298,#79299,#79300,#79301,#79302,#79303,#79304,#79305,#79306,#79307,#79308,
#79309,#79310,#79311,#79312,#79313,#79314,#79315,#79316,#79317,#79318,#79319,
#79320,#79321,#79322,#79323,#79324,#79325,#79326,#79327,#79328),
 .UNSPECIFIED.,.F.,.F.,(4,2,2,2,2,2,2,2,2,2,2,2,2,2,2,2,2,4),(-1.01710396538768,
-1.01052569025312,-0.95072976706705,-0.893102151152008,-0.833241412200572,
-0.77555546378878,-0.715629057236816,-0.657883550045956,-0.597890650662598,
-0.540084424611622,-0.480024234372677,-0.422156192345284,-0.362027940792846,
-0.304097045462937,-0.243899989848112,-0.185905260581977,-0.125638685815469,
-0.0724080849059257),.UNSPECIFIED.) ;
#1598=B_SPLINE_CURVE_WITH_KNOTS('',3,(#79330,#79331,#79332,#79333,#79334,
#79335,#79336,#79337,#79338,#79339,#79340,#79341,#79342,#79343,#79344,#79345,
#79346,#79347,#79348,#79349,#79350,#79351,#79352,#79353,#79354,#79355,#79356,
#79357,#79358,#79359,#79360,#79361,#79362,#79363,#79364,#79365),
 .UNSPECIFIED.,.F.,.F.,(4,2,2,2,2,2,2,2,2,2,2,2,2,2,2,2,2,4),(0.435597230048873,
0.495046546283641,0.565172626519024,0.632699860466232,0.702763552831684,
0.770242289348338,0.840244331880487,0.907676580521343,0.977617711024885,
1.04500561401596,1.11488656619888,1.18223240425633,1.25205390364054,1.31936010136934,
1.38912286105409,1.4563919917789,1.52609670814966,1.5389994522091),
 .UNSPECIFIED.) ;
#1599=B_SPLINE_CURVE_WITH_KNOTS('',3,(#79366,#79367,#79368,#79369,#79370,
#79371,#79372,#79373,#79374,#79375,#79376,#79377,#79378,#79379,#79380,#79381,
#79382,#79383,#79384,#79385,#79386,#79387,#79388,#79389,#79390,#79391,#79392,
#79393,#79394,#79395,#79396,#79397,#79398,#79399,#79400,#79401),
 .UNSPECIFIED.,.F.,.F.,(4,2,2,2,2,2,2,2,2,2,2,2,2,2,2,2,2,4),(2.76015985424245,
2.77763902868009,2.84767181663405,2.91539980943377,2.98548785867969,3.05323670495124,
3.12338056402631,3.1911537061991,3.26135395879188,3.32915468023334,3.39941194304139,
3.46724336682288,3.53755828661268,3.60542337583455,3.67579662590241,3.74369818538195,
3.81413046159021,3.87088446641146),.UNSPECIFIED.) ;
#1600=B_SPLINE_CURVE_WITH_KNOTS('',3,(#79532,#79533,#79534,#79535),
 .UNSPECIFIED.,.F.,.F.,(4,4),(0.,0.00842756229585243),.UNSPECIFIED.) ;
#1601=B_SPLINE_CURVE_WITH_KNOTS('',3,(#79538,#79539,#79540,#79541),
 .UNSPECIFIED.,.F.,.F.,(4,4),(0.0790172234209096,0.0874447857167618),
 .UNSPECIFIED.) ;
#1602=B_SPLINE_CURVE_WITH_KNOTS('',3,(#79588,#79589,#79590,#79591),
 .UNSPECIFIED.,.F.,.F.,(4,4),(0.,0.00842756229585143),.UNSPECIFIED.) ;
#1603=B_SPLINE_CURVE_WITH_KNOTS('',3,(#79595,#79596,#79597,#79598),
 .UNSPECIFIED.,.F.,.F.,(4,4),(0.0790172234209045,0.0874447857167594),
 .UNSPECIFIED.) ;
#1604=B_SPLINE_CURVE_WITH_KNOTS('',3,(#79639,#79640,#79641,#79642,#79643,
#79644,#79645,#79646,#79647,#79648,#79649,#79650),.UNSPECIFIED.,.F.,.F.,
(4,2,2,2,2,4),(1.00000007519743E-6,0.0421735173272767,0.08211256883264,
0.109687200675272,0.164822029616579,0.245179037282195),.UNSPECIFIED.) ;
#1605=B_SPLINE_CURVE_WITH_KNOTS('',3,(#79651,#79652,#79653,#79654,#79655,
#79656,#79657,#79658,#79659,#79660),.UNSPECIFIED.,.F.,.F.,(4,2,2,2,4),(1.0000001480151E-6,
0.0490152958922886,0.0835871661537387,0.106392725679102,0.131008894822419),
 .UNSPECIFIED.) ;
#1606=B_SPLINE_CURVE_WITH_KNOTS('',3,(#79669,#79670,#79671,#79672,#79673,
#79674,#79675,#79676,#79677,#79678,#79679,#79680),.UNSPECIFIED.,.F.,.F.,
(4,2,2,2,2,4),(-0.00017826200870649,0.,0.0030884165059787,0.00619403925206626,
0.0112943329275738,0.0143635991137086),.UNSPECIFIED.) ;
#1607=B_SPLINE_CURVE_WITH_KNOTS('',3,(#79682,#79683,#79684,#79685,#79686,
#79687,#79688,#79689,#79690,#79691,#79692,#79693),.UNSPECIFIED.,.F.,.F.,
(4,2,2,2,2,4),(0.0308002519686446,0.0338695181549982,0.0389698118306942,
0.0420754345767631,0.0451638510827407,0.045342113091339),.UNSPECIFIED.) ;
#1608=B_SPLINE_CURVE_WITH_KNOTS('',3,(#79697,#79698,#79699,#79700,#79701,
#79702,#79703,#79704,#79705,#79706,#79707,#79708),.UNSPECIFIED.,.F.,.F.,
(4,2,2,2,2,4),(0.0308002519713024,0.0338695181576853,0.0389698118335861,
0.0420754345799843,0.0451638510866813,0.0453421130955797),.UNSPECIFIED.) ;
#1609=B_SPLINE_CURVE_WITH_KNOTS('',3,(#79711,#79712,#79713,#79714,#79715,
#79716,#79717,#79718,#79719,#79720,#79721,#79722),.UNSPECIFIED.,.F.,.F.,
(4,2,2,2,2,4),(-0.000178262008688658,2.5170620795989E-14,0.00308841650593589,
0.00619403925194464,0.0112943329278571,0.0143635991142711),
 .UNSPECIFIED.) ;
#1610=B_SPLINE_CURVE_WITH_KNOTS('',3,(#79903,#79904,#79905,#79906,#79907,
#79908,#79909,#79910,#79911,#79912),.UNSPECIFIED.,.F.,.F.,(4,2,2,2,4),(1.00000014819981E-6,
0.0516668726729712,0.117271294398376,0.174520707500308,0.234084768444643),
 .UNSPECIFIED.) ;
#1611=B_SPLINE_CURVE_WITH_KNOTS('',3,(#79913,#79914,#79915,#79916,#79917,
#79918,#79919,#79920,#79921,#79922),.UNSPECIFIED.,.F.,.F.,(4,2,2,2,4),(9.99997439055519E-7,
0.0477521616236099,0.0878727120265759,0.124072211679175,0.147007126409162),
 .UNSPECIFIED.) ;
#2173=PLANE('',#35985) ;
#2174=PLANE('',#35988) ;
#2175=PLANE('',#35991) ;
#2176=PLANE('',#35992) ;
#2177=PLANE('',#35993) ;
#2178=PLANE('',#35994) ;
#2179=PLANE('',#36000) ;
#2180=PLANE('',#36003) ;
#2181=PLANE('',#36004) ;
#2182=PLANE('',#36005) ;
#2183=PLANE('',#36006) ;
#2184=PLANE('',#36009) ;
#2185=PLANE('',#36018) ;
#2186=PLANE('',#36022) ;
#2187=PLANE('',#36025) ;
#2188=PLANE('',#36031) ;
#2189=PLANE('',#36126) ;
#2190=PLANE('',#36133) ;
#3853=FACE_OUTER_BOUND('',#5911,.T.) ;
#3854=FACE_OUTER_BOUND('',#5912,.T.) ;
#3855=FACE_OUTER_BOUND('',#5913,.T.) ;
#3856=FACE_OUTER_BOUND('',#5914,.T.) ;
#3857=FACE_OUTER_BOUND('',#5915,.T.) ;
#3858=FACE_OUTER_BOUND('',#5916,.T.) ;
#3859=FACE_OUTER_BOUND('',#5917,.T.) ;
#3860=FACE_OUTER_BOUND('',#5918,.T.) ;
#3861=FACE_OUTER_BOUND('',#5919,.T.) ;
#3862=FACE_OUTER_BOUND('',#5920,.T.) ;
#3863=FACE_OUTER_BOUND('',#5921,.T.) ;
#3864=FACE_OUTER_BOUND('',#5922,.T.) ;
#3865=FACE_OUTER_BOUND('',#5923,.T.) ;
#3866=FACE_OUTER_BOUND('',#5924,.T.) ;
#3867=FACE_OUTER_BOUND('',#5925,.T.) ;
#3868=FACE_OUTER_BOUND('',#5926,.T.) ;
#3869=FACE_OUTER_BOUND('',#5927,.T.) ;
#3870=FACE_OUTER_BOUND('',#5928,.T.) ;
#3871=FACE_OUTER_BOUND('',#5929,.T.) ;
#3872=FACE_OUTER_BOUND('',#5930,.T.) ;
#3873=FACE_OUTER_BOUND('',#5931,.T.) ;
#3874=FACE_OUTER_BOUND('',#5932,.T.) ;
#3875=FACE_OUTER_BOUND('',#5933,.T.) ;
#3876=FACE_OUTER_BOUND('',#5934,.T.) ;
#3877=FACE_OUTER_BOUND('',#5935,.T.) ;
#3878=FACE_OUTER_BOUND('',#5936,.T.) ;
#3879=FACE_OUTER_BOUND('',#5937,.T.) ;
#3880=FACE_OUTER_BOUND('',#5938,.T.) ;
#3881=FACE_OUTER_BOUND('',#5939,.T.) ;
#3882=FACE_OUTER_BOUND('',#5940,.T.) ;
#3883=FACE_OUTER_BOUND('',#5941,.T.) ;
#3884=FACE_OUTER_BOUND('',#5942,.T.) ;
#3885=FACE_OUTER_BOUND('',#5943,.T.) ;
#3886=FACE_OUTER_BOUND('',#5944,.T.) ;
#3887=FACE_OUTER_BOUND('',#5945,.T.) ;
#3888=FACE_OUTER_BOUND('',#5946,.T.) ;
#3889=FACE_OUTER_BOUND('',#5947,.T.) ;
#3890=FACE_OUTER_BOUND('',#5948,.T.) ;
#3891=FACE_OUTER_BOUND('',#5949,.T.) ;
#3892=FACE_OUTER_BOUND('',#5950,.T.) ;
#3893=FACE_OUTER_BOUND('',#5951,.T.) ;
#3894=FACE_OUTER_BOUND('',#5952,.T.) ;
#3895=FACE_OUTER_BOUND('',#5953,.T.) ;
#3896=FACE_OUTER_BOUND('',#5954,.T.) ;
#3897=FACE_OUTER_BOUND('',#5955,.T.) ;
#3898=FACE_OUTER_BOUND('',#5956,.T.) ;
#3899=FACE_OUTER_BOUND('',#5957,.T.) ;
#3900=FACE_OUTER_BOUND('',#5958,.T.) ;
#3901=FACE_OUTER_BOUND('',#5959,.T.) ;
#3902=FACE_OUTER_BOUND('',#5961,.T.) ;
#3903=FACE_OUTER_BOUND('',#5962,.T.) ;
#3904=FACE_OUTER_BOUND('',#5963,.T.) ;
#3905=FACE_OUTER_BOUND('',#5964,.T.) ;
#3906=FACE_OUTER_BOUND('',#5965,.T.) ;
#3907=FACE_OUTER_BOUND('',#5966,.T.) ;
#3908=FACE_OUTER_BOUND('',#5967,.T.) ;
#3909=FACE_OUTER_BOUND('',#5968,.T.) ;
#3910=FACE_OUTER_BOUND('',#5969,.T.) ;
#3911=FACE_OUTER_BOUND('',#5970,.T.) ;
#3912=FACE_OUTER_BOUND('',#5971,.T.) ;
#3913=FACE_OUTER_BOUND('',#5972,.T.) ;
#3914=FACE_OUTER_BOUND('',#5973,.T.) ;
#3915=FACE_OUTER_BOUND('',#5974,.T.) ;
#3916=FACE_OUTER_BOUND('',#5975,.T.) ;
#3917=FACE_OUTER_BOUND('',#5976,.T.) ;
#3918=FACE_OUTER_BOUND('',#5977,.T.) ;
#3919=FACE_OUTER_BOUND('',#5978,.T.) ;
#3920=FACE_OUTER_BOUND('',#5979,.T.) ;
#3921=FACE_OUTER_BOUND('',#5980,.T.) ;
#3922=FACE_OUTER_BOUND('',#5981,.T.) ;
#3923=FACE_OUTER_BOUND('',#5982,.T.) ;
#3924=FACE_OUTER_BOUND('',#5983,.T.) ;
#3925=FACE_OUTER_BOUND('',#5984,.T.) ;
#3926=FACE_OUTER_BOUND('',#5985,.T.) ;
#3927=FACE_OUTER_BOUND('',#5986,.T.) ;
#3928=FACE_OUTER_BOUND('',#5987,.T.) ;
#3929=FACE_OUTER_BOUND('',#5988,.T.) ;
#3930=FACE_OUTER_BOUND('',#5989,.T.) ;
#3931=FACE_OUTER_BOUND('',#5990,.T.) ;
#3932=FACE_OUTER_BOUND('',#5991,.T.) ;
#3933=FACE_OUTER_BOUND('',#5992,.T.) ;
#3934=FACE_OUTER_BOUND('',#5993,.T.) ;
#3935=FACE_OUTER_BOUND('',#5994,.T.) ;
#3936=FACE_OUTER_BOUND('',#5995,.T.) ;
#3937=FACE_OUTER_BOUND('',#5996,.T.) ;
#3938=FACE_OUTER_BOUND('',#5997,.T.) ;
#3939=FACE_OUTER_BOUND('',#5998,.T.) ;
#3940=FACE_OUTER_BOUND('',#5999,.T.) ;
#3941=FACE_OUTER_BOUND('',#6000,.T.) ;
#3942=FACE_OUTER_BOUND('',#6001,.T.) ;
#3943=FACE_OUTER_BOUND('',#6002,.T.) ;
#3944=FACE_OUTER_BOUND('',#6003,.T.) ;
#3945=FACE_OUTER_BOUND('',#6004,.T.) ;
#3946=FACE_OUTER_BOUND('',#6005,.T.) ;
#3947=FACE_OUTER_BOUND('',#6006,.T.) ;
#3948=FACE_OUTER_BOUND('',#6007,.T.) ;
#3949=FACE_OUTER_BOUND('',#6008,.T.) ;
#3950=FACE_OUTER_BOUND('',#6009,.T.) ;
#3951=FACE_OUTER_BOUND('',#6010,.T.) ;
#3952=FACE_OUTER_BOUND('',#6011,.T.) ;
#3953=FACE_OUTER_BOUND('',#6012,.T.) ;
#3954=FACE_OUTER_BOUND('',#6013,.T.) ;
#3955=FACE_OUTER_BOUND('',#6014,.T.) ;
#3956=FACE_OUTER_BOUND('',#6016,.T.) ;
#3957=FACE_OUTER_BOUND('',#6017,.T.) ;
#3958=FACE_OUTER_BOUND('',#6018,.T.) ;
#3959=FACE_OUTER_BOUND('',#6020,.T.) ;
#3960=FACE_OUTER_BOUND('',#6021,.T.) ;
#5911=EDGE_LOOP('',(#28422,#28423,#28424,#28425)) ;
#5912=EDGE_LOOP('',(#28426,#28427,#28428,#28429)) ;
#5913=EDGE_LOOP('',(#28430,#28431,#28432,#28433)) ;
#5914=EDGE_LOOP('',(#28434,#28435,#28436,#28437)) ;
#5915=EDGE_LOOP('',(#28438,#28439,#28440,#28441)) ;
#5916=EDGE_LOOP('',(#28442,#28443,#28444,#28445)) ;
#5917=EDGE_LOOP('',(#28446,#28447,#28448,#28449)) ;
#5918=EDGE_LOOP('',(#28450,#28451,#28452,#28453)) ;
#5919=EDGE_LOOP('',(#28454,#28455,#28456,#28457)) ;
#5920=EDGE_LOOP('',(#28458,#28459,#28460,#28461)) ;
#5921=EDGE_LOOP('',(#28462,#28463,#28464,#28465)) ;
#5922=EDGE_LOOP('',(#28466,#28467,#28468,#28469)) ;
#5923=EDGE_LOOP('',(#28470,#28471,#28472,#28473)) ;
#5924=EDGE_LOOP('',(#28474,#28475,#28476,#28477)) ;
#5925=EDGE_LOOP('',(#28478,#28479,#28480,#28481)) ;
#5926=EDGE_LOOP('',(#28482,#28483,#28484,#28485)) ;
#5927=EDGE_LOOP('',(#28486,#28487,#28488,#28489)) ;
#5928=EDGE_LOOP('',(#28490,#28491,#28492,#28493)) ;
#5929=EDGE_LOOP('',(#28494,#28495,#28496,#28497)) ;
#5930=EDGE_LOOP('',(#28498,#28499,#28500,#28501)) ;
#5931=EDGE_LOOP('',(#28502,#28503,#28504,#28505)) ;
#5932=EDGE_LOOP('',(#28506,#28507,#28508,#28509)) ;
#5933=EDGE_LOOP('',(#28510,#28511,#28512,#28513)) ;
#5934=EDGE_LOOP('',(#28514,#28515,#28516,#28517)) ;
#5935=EDGE_LOOP('',(#28518,#28519,#28520,#28521)) ;
#5936=EDGE_LOOP('',(#28522,#28523,#28524,#28525)) ;
#5937=EDGE_LOOP('',(#28526,#28527,#28528,#28529)) ;
#5938=EDGE_LOOP('',(#28530,#28531,#28532)) ;
#5939=EDGE_LOOP('',(#28533,#28534,#28535)) ;
#5940=EDGE_LOOP('',(#28536,#28537,#28538,#28539)) ;
#5941=EDGE_LOOP('',(#28540,#28541,#28542)) ;
#5942=EDGE_LOOP('',(#28543,#28544,#28545)) ;
#5943=EDGE_LOOP('',(#28546,#28547,#28548,#28549)) ;
#5944=EDGE_LOOP('',(#28550,#28551,#28552,#28553)) ;
#5945=EDGE_LOOP('',(#28554,#28555,#28556,#28557,#28558,#28559,#28560,#28561,
#28562,#28563,#28564,#28565)) ;
#5946=EDGE_LOOP('',(#28566,#28567,#28568,#28569)) ;
#5947=EDGE_LOOP('',(#28570,#28571,#28572,#28573)) ;
#5948=EDGE_LOOP('',(#28574,#28575,#28576,#28577)) ;
#5949=EDGE_LOOP('',(#28578,#28579,#28580,#28581)) ;
#5950=EDGE_LOOP('',(#28582,#28583,#28584,#28585)) ;
#5951=EDGE_LOOP('',(#28586,#28587,#28588,#28589)) ;
#5952=EDGE_LOOP('',(#28590,#28591,#28592,#28593)) ;
#5953=EDGE_LOOP('',(#28594,#28595,#28596,#28597)) ;
#5954=EDGE_LOOP('',(#28598,#28599,#28600,#28601,#28602,#28603,#28604,#28605,
#28606,#28607,#28608,#28609,#28610,#28611,#28612,#28613)) ;
#5955=EDGE_LOOP('',(#28614,#28615,#28616,#28617)) ;
#5956=EDGE_LOOP('',(#28618,#28619,#28620,#28621,#28622,#28623)) ;
#5957=EDGE_LOOP('',(#28624,#28625,#28626,#28627)) ;
#5958=EDGE_LOOP('',(#28628,#28629,#28630,#28631,#28632,#28633,#28634,#28635,
#28636,#28637)) ;
#5959=EDGE_LOOP('',(#28638,#28639,#28640,#28641)) ;
#5960=EDGE_LOOP('',(#28642,#28643,#28644,#28645)) ;
#5961=EDGE_LOOP('',(#28646,#28647,#28648,#28649)) ;
#5962=EDGE_LOOP('',(#28650,#28651,#28652,#28653)) ;
#5963=EDGE_LOOP('',(#28654,#28655,#28656,#28657)) ;
#5964=EDGE_LOOP('',(#28658,#28659,#28660,#28661)) ;
#5965=EDGE_LOOP('',(#28662,#28663,#28664,#28665)) ;
#5966=EDGE_LOOP('',(#28666,#28667,#28668,#28669)) ;
#5967=EDGE_LOOP('',(#28670,#28671,#28672,#28673,#28674,#28675)) ;
#5968=EDGE_LOOP('',(#28676,#28677,#28678,#28679,#28680,#28681)) ;
#5969=EDGE_LOOP('',(#28682,#28683,#28684,#28685)) ;
#5970=EDGE_LOOP('',(#28686,#28687,#28688,#28689)) ;
#5971=EDGE_LOOP('',(#28690,#28691,#28692,#28693,#28694)) ;
#5972=EDGE_LOOP('',(#28695,#28696,#28697,#28698,#28699)) ;
#5973=EDGE_LOOP('',(#28700,#28701,#28702,#28703,#28704)) ;
#5974=EDGE_LOOP('',(#28705,#28706,#28707)) ;
#5975=EDGE_LOOP('',(#28708,#28709,#28710,#28711,#28712)) ;
#5976=EDGE_LOOP('',(#28713,#28714,#28715)) ;
#5977=EDGE_LOOP('',(#28716,#28717,#28718,#28719)) ;
#5978=EDGE_LOOP('',(#28720,#28721,#28722,#28723)) ;
#5979=EDGE_LOOP('',(#28724,#28725,#28726,#28727)) ;
#5980=EDGE_LOOP('',(#28728,#28729,#28730,#28731)) ;
#5981=EDGE_LOOP('',(#28732,#28733,#28734,#28735)) ;
#5982=EDGE_LOOP('',(#28736,#28737,#28738,#28739)) ;
#5983=EDGE_LOOP('',(#28740,#28741,#28742,#28743)) ;
#5984=EDGE_LOOP('',(#28744,#28745,#28746,#28747)) ;
#5985=EDGE_LOOP('',(#28748,#28749,#28750,#28751)) ;
#5986=EDGE_LOOP('',(#28752,#28753,#28754,#28755)) ;
#5987=EDGE_LOOP('',(#28756,#28757,#28758,#28759)) ;
#5988=EDGE_LOOP('',(#28760,#28761,#28762,#28763)) ;
#5989=EDGE_LOOP('',(#28764,#28765,#28766,#28767)) ;
#5990=EDGE_LOOP('',(#28768,#28769,#28770,#28771)) ;
#5991=EDGE_LOOP('',(#28772,#28773,#28774,#28775)) ;
#5992=EDGE_LOOP('',(#28776,#28777,#28778,#28779)) ;
#5993=EDGE_LOOP('',(#28780,#28781,#28782,#28783)) ;
#5994=EDGE_LOOP('',(#28784,#28785,#28786,#28787)) ;
#5995=EDGE_LOOP('',(#28788,#28789,#28790,#28791)) ;
#5996=EDGE_LOOP('',(#28792,#28793,#28794,#28795)) ;
#5997=EDGE_LOOP('',(#28796,#28797,#28798,#28799)) ;
#5998=EDGE_LOOP('',(#28800,#28801,#28802,#28803)) ;
#5999=EDGE_LOOP('',(#28804,#28805,#28806,#28807)) ;
#6000=EDGE_LOOP('',(#28808,#28809,#28810)) ;
#6001=EDGE_LOOP('',(#28811,#28812,#28813)) ;
#6002=EDGE_LOOP('',(#28814,#28815,#28816,#28817)) ;
#6003=EDGE_LOOP('',(#28818,#28819,#28820,#28821)) ;
#6004=EDGE_LOOP('',(#28822,#28823,#28824,#28825)) ;
#6005=EDGE_LOOP('',(#28826,#28827,#28828,#28829)) ;
#6006=EDGE_LOOP('',(#28830,#28831,#28832,#28833)) ;
#6007=EDGE_LOOP('',(#28834,#28835,#28836)) ;
#6008=EDGE_LOOP('',(#28837,#28838,#28839)) ;
#6009=EDGE_LOOP('',(#28840,#28841,#28842)) ;
#6010=EDGE_LOOP('',(#28843,#28844,#28845)) ;
#6011=EDGE_LOOP('',(#28846,#28847,#28848,#28849)) ;
#6012=EDGE_LOOP('',(#28850,#28851,#28852,#28853)) ;
#6013=EDGE_LOOP('',(#28854,#28855,#28856,#28857)) ;
#6014=EDGE_LOOP('',(#28858,#28859,#28860,#28861,#28862,#28863,#28864,#28865,
#28866,#28867,#28868,#28869,#28870,#28871,#28872,#28873)) ;
#6015=EDGE_LOOP('',(#28874)) ;
#6016=EDGE_LOOP('',(#28875,#28876,#28877,#28878,#28879)) ;
#6017=EDGE_LOOP('',(#28880,#28881,#28882,#28883,#28884)) ;
#6018=EDGE_LOOP('',(#28885)) ;
#6019=EDGE_LOOP('',(#28886,#28887,#28888,#28889)) ;
#6020=EDGE_LOOP('',(#28890,#28891,#28892,#28893,#28894,#28895,#28896,#28897,
#28898,#28899,#28900,#28901)) ;
#6021=EDGE_LOOP('',(#28902,#28903,#28904,#28905,#28906,#28907,#28908,#28909,
#28910,#28911,#28912,#28913)) ;
#8197=LINE('',#78791,#10516) ;
#8198=LINE('',#78834,#10517) ;
#8199=LINE('',#78910,#10518) ;
#8200=LINE('',#78986,#10519) ;
#8201=LINE('',#79025,#10520) ;
#8202=LINE('',#79068,#10521) ;
#8203=LINE('',#79144,#10522) ;
#8204=LINE('',#79220,#10523) ;
#8205=LINE('',#79407,#10524) ;
#8206=LINE('',#79410,#10525) ;
#8207=LINE('',#79424,#10526) ;
#8208=LINE('',#79425,#10527) ;
#8209=LINE('',#79448,#10528) ;
#8210=LINE('',#79449,#10529) ;
#8211=LINE('',#79457,#10530) ;
#8212=LINE('',#79458,#10531) ;
#8213=LINE('',#79462,#10532) ;
#8214=LINE('',#79463,#10533) ;
#8215=LINE('',#79476,#10534) ;
#8216=LINE('',#79477,#10535) ;
#8217=LINE('',#79482,#10536) ;
#8218=LINE('',#79483,#10537) ;
#8219=LINE('',#79491,#10538) ;
#8220=LINE('',#79492,#10539) ;
#8221=LINE('',#79494,#10540) ;
#8222=LINE('',#79495,#10541) ;
#8223=LINE('',#79500,#10542) ;
#8224=LINE('',#79501,#10543) ;
#8225=LINE('',#79503,#10544) ;
#8226=LINE('',#79504,#10545) ;
#8227=LINE('',#79513,#10546) ;
#8228=LINE('',#79515,#10547) ;
#8229=LINE('',#79521,#10548) ;
#8230=LINE('',#79524,#10549) ;
#8231=LINE('',#79527,#10550) ;
#8232=LINE('',#79530,#10551) ;
#8233=LINE('',#79537,#10552) ;
#8234=LINE('',#79544,#10553) ;
#8235=LINE('',#79548,#10554) ;
#8236=LINE('',#79549,#10555) ;
#8237=LINE('',#79553,#10556) ;
#8238=LINE('',#79557,#10557) ;
#8239=LINE('',#79561,#10558) ;
#8240=LINE('',#79564,#10559) ;
#8241=LINE('',#79569,#10560) ;
#8242=LINE('',#79571,#10561) ;
#8243=LINE('',#79573,#10562) ;
#8244=LINE('',#79575,#10563) ;
#8245=LINE('',#79577,#10564) ;
#8246=LINE('',#79580,#10565) ;
#8247=LINE('',#79584,#10566) ;
#8248=LINE('',#79586,#10567) ;
#8249=LINE('',#79593,#10568) ;
#8250=LINE('',#79599,#10569) ;
#8251=LINE('',#79603,#10570) ;
#8252=LINE('',#79605,#10571) ;
#8253=LINE('',#79607,#10572) ;
#8254=LINE('',#79608,#10573) ;
#8255=LINE('',#79612,#10574) ;
#8256=LINE('',#79614,#10575) ;
#8257=LINE('',#79618,#10576) ;
#8258=LINE('',#79620,#10577) ;
#8259=LINE('',#79622,#10578) ;
#8260=LINE('',#79624,#10579) ;
#8261=LINE('',#79626,#10580) ;
#8262=LINE('',#79629,#10581) ;
#8263=LINE('',#79633,#10582) ;
#8264=LINE('',#79635,#10583) ;
#8265=LINE('',#79637,#10584) ;
#8266=LINE('',#79638,#10585) ;
#8267=LINE('',#79694,#10586) ;
#8268=LINE('',#79710,#10587) ;
#8269=LINE('',#79726,#10588) ;
#8270=LINE('',#79728,#10589) ;
#8271=LINE('',#79730,#10590) ;
#8272=LINE('',#79731,#10591) ;
#8273=LINE('',#79738,#10592) ;
#8274=LINE('',#79740,#10593) ;
#8275=LINE('',#79744,#10594) ;
#8276=LINE('',#79747,#10595) ;
#8277=LINE('',#79751,#10596) ;
#8278=LINE('',#79755,#10597) ;
#8279=LINE('',#79759,#10598) ;
#8280=LINE('',#79760,#10599) ;
#8281=LINE('',#79765,#10600) ;
#8282=LINE('',#79769,#10601) ;
#8283=LINE('',#79771,#10602) ;
#8284=LINE('',#79772,#10603) ;
#8285=LINE('',#79799,#10604) ;
#8286=LINE('',#79802,#10605) ;
#8287=LINE('',#79807,#10606) ;
#8288=LINE('',#79812,#10607) ;
#8289=LINE('',#79828,#10608) ;
#8290=LINE('',#79833,#10609) ;
#8291=LINE('',#79848,#10610) ;
#8292=LINE('',#79868,#10611) ;
#8293=LINE('',#79871,#10612) ;
#8294=LINE('',#79876,#10613) ;
#8295=LINE('',#79899,#10614) ;
#10516=VECTOR('',#44771,1.7526) ;
#10517=VECTOR('',#44776,1.7526) ;
#10518=VECTOR('',#44779,1.7526) ;
#10519=VECTOR('',#44782,1.7526) ;
#10520=VECTOR('',#44787,1.5) ;
#10521=VECTOR('',#44792,1.5) ;
#10522=VECTOR('',#44795,1.5) ;
#10523=VECTOR('',#44798,1.5) ;
#10524=VECTOR('',#44809,10.) ;
#10525=VECTOR('',#44812,10.) ;
#10526=VECTOR('',#44827,10.) ;
#10527=VECTOR('',#44828,10.) ;
#10528=VECTOR('',#44853,10.) ;
#10529=VECTOR('',#44854,10.) ;
#10530=VECTOR('',#44865,10.) ;
#10531=VECTOR('',#44866,10.) ;
#10532=VECTOR('',#44871,10.) ;
#10533=VECTOR('',#44872,10.) ;
#10534=VECTOR('',#44887,10.) ;
#10535=VECTOR('',#44888,10.) ;
#10536=VECTOR('',#44893,10.) ;
#10537=VECTOR('',#44894,10.) ;
#10538=VECTOR('',#44905,10.) ;
#10539=VECTOR('',#44906,10.) ;
#10540=VECTOR('',#44909,10.) ;
#10541=VECTOR('',#44910,10.) ;
#10542=VECTOR('',#44915,10.) ;
#10543=VECTOR('',#44916,10.) ;
#10544=VECTOR('',#44919,10.) ;
#10545=VECTOR('',#44920,10.) ;
#10546=VECTOR('',#44933,10.) ;
#10547=VECTOR('',#44936,10.) ;
#10548=VECTOR('',#44947,6.35) ;
#10549=VECTOR('',#44950,10.) ;
#10550=VECTOR('',#44953,0.125) ;
#10551=VECTOR('',#44956,10.) ;
#10552=VECTOR('',#44957,6.35) ;
#10553=VECTOR('',#44960,10.) ;
#10554=VECTOR('',#44965,10.) ;
#10555=VECTOR('',#44966,10.) ;
#10556=VECTOR('',#44973,6.35) ;
#10557=VECTOR('',#44978,10.) ;
#10558=VECTOR('',#44983,10.) ;
#10559=VECTOR('',#44986,10.) ;
#10560=VECTOR('',#44991,10.) ;
#10561=VECTOR('',#44992,10.) ;
#10562=VECTOR('',#44993,6.35) ;
#10563=VECTOR('',#44994,10.) ;
#10564=VECTOR('',#44995,10.) ;
#10565=VECTOR('',#45000,10.) ;
#10566=VECTOR('',#45003,10.) ;
#10567=VECTOR('',#45004,10.) ;
#10568=VECTOR('',#45005,6.35) ;
#10569=VECTOR('',#45006,10.) ;
#10570=VECTOR('',#45009,10.) ;
#10571=VECTOR('',#45010,10.) ;
#10572=VECTOR('',#45011,10.) ;
#10573=VECTOR('',#45012,10.) ;
#10574=VECTOR('',#45015,10.) ;
#10575=VECTOR('',#45016,10.) ;
#10576=VECTOR('',#45019,10.) ;
#10577=VECTOR('',#45020,10.) ;
#10578=VECTOR('',#45021,6.35) ;
#10579=VECTOR('',#45022,10.) ;
#10580=VECTOR('',#45023,10.) ;
#10581=VECTOR('',#45026,10.) ;
#10582=VECTOR('',#45029,10.) ;
#10583=VECTOR('',#45030,6.35) ;
#10584=VECTOR('',#45031,10.) ;
#10585=VECTOR('',#45032,6.35) ;
#10586=VECTOR('',#45047,10.) ;
#10587=VECTOR('',#45050,10.) ;
#10588=VECTOR('',#45053,10.) ;
#10589=VECTOR('',#45054,10.) ;
#10590=VECTOR('',#45055,10.) ;
#10591=VECTOR('',#45056,10.) ;
#10592=VECTOR('',#45065,10.) ;
#10593=VECTOR('',#45066,10.) ;
#10594=VECTOR('',#45069,10.) ;
#10595=VECTOR('',#45072,10.) ;
#10596=VECTOR('',#45075,10.) ;
#10597=VECTOR('',#45078,10.) ;
#10598=VECTOR('',#45081,10.) ;
#10599=VECTOR('',#45082,10.) ;
#10600=VECTOR('',#45087,10.) ;
#10601=VECTOR('',#45092,10.) ;
#10602=VECTOR('',#45093,10.) ;
#10603=VECTOR('',#45094,10.) ;
#10604=VECTOR('',#45137,10.) ;
#10605=VECTOR('',#45140,10.) ;
#10606=VECTOR('',#45147,10.) ;
#10607=VECTOR('',#45154,10.) ;
#10608=VECTOR('',#45183,10.) ;
#10609=VECTOR('',#45190,10.) ;
#10610=VECTOR('',#45217,10.) ;
#10611=VECTOR('',#45254,10.) ;
#10612=VECTOR('',#45259,10.) ;
#10613=VECTOR('',#45268,10.) ;
#10614=VECTOR('',#45303,2.8575) ;
#12396=CIRCLE('',#35914,1.7526) ;
#12397=CIRCLE('',#35918,1.7526) ;
#12398=CIRCLE('',#35920,1.5) ;
#12399=CIRCLE('',#35924,1.5) ;
#12400=CIRCLE('',#35928,0.124999999999993) ;
#12401=CIRCLE('',#35929,0.124999999999993) ;
#12402=CIRCLE('',#35931,0.0634999999999941) ;
#12403=CIRCLE('',#35932,0.124999999999993) ;
#12404=CIRCLE('',#35933,0.188499999999987) ;
#12405=CIRCLE('',#35934,0.124999999999993) ;
#12406=CIRCLE('',#35936,0.124999999999993) ;
#12407=CIRCLE('',#35938,0.0634999999999764) ;
#12408=CIRCLE('',#35939,0.124999999999957) ;
#12409=CIRCLE('',#35940,0.188499999999969) ;
#12410=CIRCLE('',#35941,0.124999999999993) ;
#12411=CIRCLE('',#35943,0.0634999999999941) ;
#12412=CIRCLE('',#35944,0.124999999999993) ;
#12413=CIRCLE('',#35945,0.188499999999987) ;
#12414=CIRCLE('',#35946,0.124999999999993) ;
#12415=CIRCLE('',#35948,0.124999999999975) ;
#12416=CIRCLE('',#35950,0.124999999999851) ;
#12417=CIRCLE('',#35951,0.509999999999996) ;
#12418=CIRCLE('',#35952,0.634999999999996) ;
#12419=CIRCLE('',#35955,0.125000000000028) ;
#12420=CIRCLE('',#35957,0.0634999999999941) ;
#12421=CIRCLE('',#35958,0.124999999999993) ;
#12422=CIRCLE('',#35959,0.188499999999987) ;
#12423=CIRCLE('',#35960,0.124999999999993) ;
#12424=CIRCLE('',#35962,0.124999999999993) ;
#12425=CIRCLE('',#35964,0.125000000000064) ;
#12426=CIRCLE('',#35966,0.125000000000099) ;
#12427=CIRCLE('',#35967,0.509999999999996) ;
#12428=CIRCLE('',#35968,0.634999999999996) ;
#12429=CIRCLE('',#35972,0.124999999999993) ;
#12430=CIRCLE('',#35975,0.124999999999993) ;
#12431=CIRCLE('',#35977,0.124999999999993) ;
#12432=CIRCLE('',#35979,0.124999999999993) ;
#12433=CIRCLE('',#35980,0.124999999999993) ;
#12434=CIRCLE('',#35982,0.124999999999993) ;
#12435=CIRCLE('',#35984,0.124999999999993) ;
#12436=CIRCLE('',#35987,0.125) ;
#12437=CIRCLE('',#35990,0.125) ;
#12438=CIRCLE('',#35997,0.124999999999993) ;
#12439=CIRCLE('',#35999,0.124999999999993) ;
#12440=CIRCLE('',#36001,0.250000000000012) ;
#12441=CIRCLE('',#36002,0.249999999999986) ;
#12442=CIRCLE('',#36007,0.249999999999995) ;
#12443=CIRCLE('',#36008,0.249999999999986) ;
#12444=CIRCLE('',#36011,0.698499999999999) ;
#12445=CIRCLE('',#36012,0.698499999999999) ;
#12446=CIRCLE('',#36014,0.698500000000001) ;
#12447=CIRCLE('',#36015,0.6985) ;
#12448=CIRCLE('',#36020,0.124999999999993) ;
#12449=CIRCLE('',#36021,0.125) ;
#12450=CIRCLE('',#36023,0.573500000000001) ;
#12451=CIRCLE('',#36024,0.573499999999999) ;
#12452=CIRCLE('',#36026,0.573499999999999) ;
#12453=CIRCLE('',#36027,0.573500000000001) ;
#12454=CIRCLE('',#36029,0.125000000000006) ;
#12455=CIRCLE('',#36030,0.125) ;
#12456=CIRCLE('',#36033,0.125000000000002) ;
#12457=CIRCLE('',#36034,0.25) ;
#12458=CIRCLE('',#36036,0.25) ;
#12459=CIRCLE('',#36037,0.124999999999993) ;
#12460=CIRCLE('',#36039,0.25) ;
#12461=CIRCLE('',#36040,0.125000000000011) ;
#12462=CIRCLE('',#36042,0.124999999999993) ;
#12463=CIRCLE('',#36043,0.125000000000011) ;
#12464=CIRCLE('',#36045,0.125000000000002) ;
#12465=CIRCLE('',#36046,0.25) ;
#12466=CIRCLE('',#36048,0.124999999999993) ;
#12467=CIRCLE('',#36049,0.125000000000002) ;
#12468=CIRCLE('',#36052,0.124999999999993) ;
#12469=CIRCLE('',#36054,0.125000000000002) ;
#12470=CIRCLE('',#36056,0.124999999999993) ;
#12471=CIRCLE('',#36057,0.125000000000011) ;
#12472=CIRCLE('',#36059,0.124999999999993) ;
#12473=CIRCLE('',#36060,0.125000000000011) ;
#12474=CIRCLE('',#36062,0.124999999999993) ;
#12475=CIRCLE('',#36063,0.124999999999993) ;
#12476=CIRCLE('',#36065,0.125000000000002) ;
#12477=CIRCLE('',#36067,0.125000000000002) ;
#12478=CIRCLE('',#36069,0.124999999999957) ;
#12479=CIRCLE('',#36071,0.124999999999975) ;
#12480=CIRCLE('',#36073,0.124999999999993) ;
#12481=CIRCLE('',#36074,0.124999999999993) ;
#12482=CIRCLE('',#36076,0.124999999999993) ;
#12483=CIRCLE('',#36077,0.125000000000002) ;
#12484=CIRCLE('',#36079,0.124999999999993) ;
#12485=CIRCLE('',#36080,0.124999999999993) ;
#12486=CIRCLE('',#36082,0.124999999999993) ;
#12487=CIRCLE('',#36084,0.125000000000011) ;
#12488=CIRCLE('',#36086,0.124999999999957) ;
#12489=CIRCLE('',#36088,0.125000000000011) ;
#12490=CIRCLE('',#36090,0.125000000000002) ;
#12491=CIRCLE('',#36092,0.124999999999993) ;
#12492=CIRCLE('',#36093,0.124999999999993) ;
#12493=CIRCLE('',#36095,0.124999999999993) ;
#12494=CIRCLE('',#36097,0.125000000000011) ;
#12495=CIRCLE('',#36099,0.124999999999993) ;
#12496=CIRCLE('',#36100,0.124999999999993) ;
#12497=CIRCLE('',#36102,0.125000000000011) ;
#12498=CIRCLE('',#36103,0.124999999999993) ;
#12499=CIRCLE('',#36107,0.124999999999993) ;
#12500=CIRCLE('',#36109,0.124999999999993) ;
#12501=CIRCLE('',#36110,0.124999999999993) ;
#12502=CIRCLE('',#36113,0.124999999999993) ;
#12503=CIRCLE('',#36114,0.124999999999993) ;
#12504=CIRCLE('',#36123,2.7325) ;
#12505=CIRCLE('',#36124,0.125) ;
#12506=CIRCLE('',#36125,2.8575) ;
#12507=CIRCLE('',#36127,2.9825) ;
#12508=CIRCLE('',#36129,2.8575) ;
#12509=CIRCLE('',#36130,2.8575) ;
#12510=CIRCLE('',#36132,0.125) ;
#15123=VERTEX_POINT('',#78789) ;
#15124=VERTEX_POINT('',#78790) ;
#15125=VERTEX_POINT('',#78792) ;
#15126=VERTEX_POINT('',#78809) ;
#15127=VERTEX_POINT('',#78832) ;
#15128=VERTEX_POINT('',#78833) ;
#15129=VERTEX_POINT('',#78908) ;
#15130=VERTEX_POINT('',#78909) ;
#15131=VERTEX_POINT('',#78984) ;
#15132=VERTEX_POINT('',#78985) ;
#15133=VERTEX_POINT('',#78987) ;
#15134=VERTEX_POINT('',#79002) ;
#15135=VERTEX_POINT('',#79023) ;
#15136=VERTEX_POINT('',#79024) ;
#15137=VERTEX_POINT('',#79026) ;
#15138=VERTEX_POINT('',#79037) ;
#15139=VERTEX_POINT('',#79066) ;
#15140=VERTEX_POINT('',#79067) ;
#15141=VERTEX_POINT('',#79142) ;
#15142=VERTEX_POINT('',#79143) ;
#15143=VERTEX_POINT('',#79218) ;
#15144=VERTEX_POINT('',#79219) ;
#15145=VERTEX_POINT('',#79221) ;
#15146=VERTEX_POINT('',#79230) ;
#15147=VERTEX_POINT('',#79403) ;
#15148=VERTEX_POINT('',#79404) ;
#15149=VERTEX_POINT('',#79406) ;
#15150=VERTEX_POINT('',#79408) ;
#15151=VERTEX_POINT('',#79412) ;
#15152=VERTEX_POINT('',#79413) ;
#15153=VERTEX_POINT('',#79415) ;
#15154=VERTEX_POINT('',#79417) ;
#15155=VERTEX_POINT('',#79421) ;
#15156=VERTEX_POINT('',#79422) ;
#15157=VERTEX_POINT('',#79427) ;
#15158=VERTEX_POINT('',#79428) ;
#15159=VERTEX_POINT('',#79430) ;
#15160=VERTEX_POINT('',#79432) ;
#15161=VERTEX_POINT('',#79436) ;
#15162=VERTEX_POINT('',#79437) ;
#15163=VERTEX_POINT('',#79439) ;
#15164=VERTEX_POINT('',#79441) ;
#15165=VERTEX_POINT('',#79445) ;
#15166=VERTEX_POINT('',#79446) ;
#15167=VERTEX_POINT('',#79451) ;
#15168=VERTEX_POINT('',#79452) ;
#15169=VERTEX_POINT('',#79460) ;
#15170=VERTEX_POINT('',#79465) ;
#15171=VERTEX_POINT('',#79466) ;
#15172=VERTEX_POINT('',#79468) ;
#15173=VERTEX_POINT('',#79470) ;
#15174=VERTEX_POINT('',#79474) ;
#15175=VERTEX_POINT('',#79479) ;
#15176=VERTEX_POINT('',#79480) ;
#15177=VERTEX_POINT('',#79485) ;
#15178=VERTEX_POINT('',#79486) ;
#15179=VERTEX_POINT('',#79497) ;
#15180=VERTEX_POINT('',#79498) ;
#15181=VERTEX_POINT('',#79510) ;
#15182=VERTEX_POINT('',#79512) ;
#15183=VERTEX_POINT('',#79523) ;
#15184=VERTEX_POINT('',#79525) ;
#15185=VERTEX_POINT('',#79529) ;
#15186=VERTEX_POINT('',#79531) ;
#15187=VERTEX_POINT('',#79536) ;
#15188=VERTEX_POINT('',#79543) ;
#15189=VERTEX_POINT('',#79547) ;
#15190=VERTEX_POINT('',#79556) ;
#15191=VERTEX_POINT('',#79560) ;
#15192=VERTEX_POINT('',#79562) ;
#15193=VERTEX_POINT('',#79566) ;
#15194=VERTEX_POINT('',#79568) ;
#15195=VERTEX_POINT('',#79570) ;
#15196=VERTEX_POINT('',#79572) ;
#15197=VERTEX_POINT('',#79574) ;
#15198=VERTEX_POINT('',#79576) ;
#15199=VERTEX_POINT('',#79582) ;
#15200=VERTEX_POINT('',#79583) ;
#15201=VERTEX_POINT('',#79585) ;
#15202=VERTEX_POINT('',#79587) ;
#15203=VERTEX_POINT('',#79592) ;
#15204=VERTEX_POINT('',#79594) ;
#15205=VERTEX_POINT('',#79601) ;
#15206=VERTEX_POINT('',#79602) ;
#15207=VERTEX_POINT('',#79604) ;
#15208=VERTEX_POINT('',#79606) ;
#15209=VERTEX_POINT('',#79610) ;
#15210=VERTEX_POINT('',#79611) ;
#15211=VERTEX_POINT('',#79613) ;
#15212=VERTEX_POINT('',#79615) ;
#15213=VERTEX_POINT('',#79617) ;
#15214=VERTEX_POINT('',#79619) ;
#15215=VERTEX_POINT('',#79621) ;
#15216=VERTEX_POINT('',#79623) ;
#15217=VERTEX_POINT('',#79625) ;
#15218=VERTEX_POINT('',#79627) ;
#15219=VERTEX_POINT('',#79631) ;
#15220=VERTEX_POINT('',#79632) ;
#15221=VERTEX_POINT('',#79634) ;
#15222=VERTEX_POINT('',#79636) ;
#15223=VERTEX_POINT('',#79668) ;
#15224=VERTEX_POINT('',#79681) ;
#15225=VERTEX_POINT('',#79696) ;
#15226=VERTEX_POINT('',#79709) ;
#15227=VERTEX_POINT('',#79724) ;
#15228=VERTEX_POINT('',#79725) ;
#15229=VERTEX_POINT('',#79727) ;
#15230=VERTEX_POINT('',#79729) ;
#15231=VERTEX_POINT('',#79736) ;
#15232=VERTEX_POINT('',#79737) ;
#15233=VERTEX_POINT('',#79739) ;
#15234=VERTEX_POINT('',#79741) ;
#15235=VERTEX_POINT('',#79743) ;
#15236=VERTEX_POINT('',#79745) ;
#15237=VERTEX_POINT('',#79749) ;
#15238=VERTEX_POINT('',#79750) ;
#15239=VERTEX_POINT('',#79752) ;
#15240=VERTEX_POINT('',#79754) ;
#15241=VERTEX_POINT('',#79756) ;
#15242=VERTEX_POINT('',#79758) ;
#15243=VERTEX_POINT('',#79762) ;
#15244=VERTEX_POINT('',#79764) ;
#15245=VERTEX_POINT('',#79768) ;
#15246=VERTEX_POINT('',#79770) ;
#15247=VERTEX_POINT('',#79774) ;
#15248=VERTEX_POINT('',#79778) ;
#15249=VERTEX_POINT('',#79782) ;
#15250=VERTEX_POINT('',#79789) ;
#15251=VERTEX_POINT('',#79797) ;
#15252=VERTEX_POINT('',#79801) ;
#15253=VERTEX_POINT('',#79805) ;
#15254=VERTEX_POINT('',#79811) ;
#15255=VERTEX_POINT('',#79826) ;
#15256=VERTEX_POINT('',#79832) ;
#15257=VERTEX_POINT('',#79847) ;
#15258=VERTEX_POINT('',#79866) ;
#15259=VERTEX_POINT('',#79886) ;
#15260=VERTEX_POINT('',#79888) ;
#15261=VERTEX_POINT('',#79892) ;
#15262=VERTEX_POINT('',#79895) ;
#15263=VERTEX_POINT('',#79896) ;
#19617=EDGE_CURVE('',#15123,#15124,#8197,.T.) ;
#19618=EDGE_CURVE('',#15124,#15125,#1580,.T.) ;
#19619=EDGE_CURVE('',#15126,#15125,#12396,.T.) ;
#19620=EDGE_CURVE('',#15123,#15126,#1581,.F.) ;
#19621=EDGE_CURVE('',#15127,#15128,#8198,.T.) ;
#19622=EDGE_CURVE('',#15128,#15124,#1582,.T.) ;
#19623=EDGE_CURVE('',#15127,#15123,#1583,.F.) ;
#19624=EDGE_CURVE('',#15129,#15130,#8199,.T.) ;
#19625=EDGE_CURVE('',#15130,#15128,#1584,.T.) ;
#19626=EDGE_CURVE('',#15129,#15127,#1585,.F.) ;
#19627=EDGE_CURVE('',#15131,#15132,#8200,.T.) ;
#19628=EDGE_CURVE('',#15133,#15131,#1586,.F.) ;
#19629=EDGE_CURVE('',#15134,#15133,#12397,.T.) ;
#19630=EDGE_CURVE('',#15134,#15132,#1587,.T.) ;
#19631=EDGE_CURVE('',#15135,#15136,#8201,.T.) ;
#19632=EDGE_CURVE('',#15136,#15137,#1588,.T.) ;
#19633=EDGE_CURVE('',#15138,#15137,#12398,.F.) ;
#19634=EDGE_CURVE('',#15138,#15135,#1589,.T.) ;
#19635=EDGE_CURVE('',#15139,#15140,#8202,.T.) ;
#19636=EDGE_CURVE('',#15140,#15136,#1590,.T.) ;
#19637=EDGE_CURVE('',#15135,#15139,#1591,.T.) ;
#19638=EDGE_CURVE('',#15141,#15142,#8203,.T.) ;
#19639=EDGE_CURVE('',#15142,#15140,#1592,.T.) ;
#19640=EDGE_CURVE('',#15139,#15141,#1593,.T.) ;
#19641=EDGE_CURVE('',#15143,#15144,#8204,.T.) ;
#19642=EDGE_CURVE('',#15143,#15145,#1594,.T.) ;
#19643=EDGE_CURVE('',#15146,#15145,#12399,.F.) ;
#19644=EDGE_CURVE('',#15146,#15144,#1595,.T.) ;
#19645=EDGE_CURVE('',#15144,#15142,#1596,.T.) ;
#19646=EDGE_CURVE('',#15141,#15143,#1597,.T.) ;
#19647=EDGE_CURVE('',#15132,#15130,#1598,.T.) ;
#19648=EDGE_CURVE('',#15131,#15129,#1599,.F.) ;
#19649=EDGE_CURVE('',#15147,#15148,#12400,.T.) ;
#19650=EDGE_CURVE('',#15148,#15149,#8205,.T.) ;
#19651=EDGE_CURVE('',#15149,#15150,#12401,.T.) ;
#19652=EDGE_CURVE('',#15150,#15147,#8206,.T.) ;
#19653=EDGE_CURVE('',#15151,#15152,#12402,.F.) ;
#19654=EDGE_CURVE('',#15153,#15151,#12403,.T.) ;
#19655=EDGE_CURVE('',#15153,#15154,#12404,.T.) ;
#19656=EDGE_CURVE('',#15152,#15154,#12405,.T.) ;
#19657=EDGE_CURVE('',#15155,#15156,#12406,.T.) ;
#19658=EDGE_CURVE('',#15156,#15153,#8207,.T.) ;
#19659=EDGE_CURVE('',#15151,#15155,#8208,.T.) ;
#19660=EDGE_CURVE('',#15157,#15158,#12407,.F.) ;
#19661=EDGE_CURVE('',#15159,#15157,#12408,.T.) ;
#19662=EDGE_CURVE('',#15159,#15160,#12409,.T.) ;
#19663=EDGE_CURVE('',#15158,#15160,#12410,.T.) ;
#19664=EDGE_CURVE('',#15161,#15162,#12411,.F.) ;
#19665=EDGE_CURVE('',#15163,#15161,#12412,.T.) ;
#19666=EDGE_CURVE('',#15163,#15164,#12413,.T.) ;
#19667=EDGE_CURVE('',#15162,#15164,#12414,.T.) ;
#19668=EDGE_CURVE('',#15165,#15166,#12415,.T.) ;
#19669=EDGE_CURVE('',#15166,#15163,#8209,.T.) ;
#19670=EDGE_CURVE('',#15161,#15165,#8210,.T.) ;
#19671=EDGE_CURVE('',#15167,#15168,#12416,.T.) ;
#19672=EDGE_CURVE('',#15168,#15166,#12417,.T.) ;
#19673=EDGE_CURVE('',#15165,#15167,#12418,.T.) ;
#19674=EDGE_CURVE('',#15154,#15168,#8211,.T.) ;
#19675=EDGE_CURVE('',#15167,#15152,#8212,.T.) ;
#19676=EDGE_CURVE('',#15169,#15149,#12419,.T.) ;
#19677=EDGE_CURVE('',#15149,#15162,#8213,.T.) ;
#19678=EDGE_CURVE('',#15164,#15169,#8214,.T.) ;
#19679=EDGE_CURVE('',#15170,#15171,#12420,.F.) ;
#19680=EDGE_CURVE('',#15172,#15170,#12421,.T.) ;
#19681=EDGE_CURVE('',#15172,#15173,#12422,.T.) ;
#19682=EDGE_CURVE('',#15171,#15173,#12423,.T.) ;
#19683=EDGE_CURVE('',#15148,#15174,#12424,.T.) ;
#19684=EDGE_CURVE('',#15174,#15172,#8215,.T.) ;
#19685=EDGE_CURVE('',#15170,#15148,#8216,.T.) ;
#19686=EDGE_CURVE('',#15175,#15176,#12425,.T.) ;
#19687=EDGE_CURVE('',#15176,#15159,#8217,.T.) ;
#19688=EDGE_CURVE('',#15157,#15175,#8218,.T.) ;
#19689=EDGE_CURVE('',#15177,#15178,#12426,.T.) ;
#19690=EDGE_CURVE('',#15178,#15176,#12427,.T.) ;
#19691=EDGE_CURVE('',#15175,#15177,#12428,.T.) ;
#19692=EDGE_CURVE('',#15173,#15178,#8219,.T.) ;
#19693=EDGE_CURVE('',#15177,#15171,#8220,.T.) ;
#19694=EDGE_CURVE('',#15171,#15161,#8221,.T.) ;
#19695=EDGE_CURVE('',#15162,#15170,#8222,.T.) ;
#19696=EDGE_CURVE('',#15179,#15180,#12429,.T.) ;
#19697=EDGE_CURVE('',#15180,#15158,#8223,.T.) ;
#19698=EDGE_CURVE('',#15160,#15179,#8224,.T.) ;
#19699=EDGE_CURVE('',#15152,#15157,#8225,.T.) ;
#19700=EDGE_CURVE('',#15158,#15151,#8226,.T.) ;
#19701=EDGE_CURVE('',#15147,#15174,#12430,.T.) ;
#19702=EDGE_CURVE('',#15169,#15150,#12431,.T.) ;
#19703=EDGE_CURVE('',#15180,#15181,#12432,.T.) ;
#19704=EDGE_CURVE('',#15181,#15182,#8227,.T.) ;
#19705=EDGE_CURVE('',#15182,#15155,#12433,.T.) ;
#19706=EDGE_CURVE('',#15155,#15180,#8228,.T.) ;
#19707=EDGE_CURVE('',#15179,#15181,#12434,.T.) ;
#19708=EDGE_CURVE('',#15182,#15156,#12435,.T.) ;
#19709=EDGE_CURVE('',#15177,#15165,#8229,.T.) ;
#19710=EDGE_CURVE('',#15169,#15183,#8230,.T.) ;
#19711=EDGE_CURVE('',#15184,#15183,#12436,.T.) ;
#19712=EDGE_CURVE('',#15150,#15184,#8231,.T.) ;
#19713=EDGE_CURVE('',#15185,#15156,#8232,.T.) ;
#19714=EDGE_CURVE('',#15185,#15186,#1600,.T.) ;
#19715=EDGE_CURVE('',#15187,#15186,#8233,.T.) ;
#19716=EDGE_CURVE('',#15187,#15183,#1601,.T.) ;
#19717=EDGE_CURVE('',#15182,#15188,#8234,.T.) ;
#19718=EDGE_CURVE('',#15185,#15188,#12437,.T.) ;
#19719=EDGE_CURVE('',#15189,#15181,#8235,.T.) ;
#19720=EDGE_CURVE('',#15188,#15189,#8236,.T.) ;
#19721=EDGE_CURVE('',#15175,#15167,#8237,.T.) ;
#19722=EDGE_CURVE('',#15179,#15190,#8238,.T.) ;
#19723=EDGE_CURVE('',#15190,#15189,#12438,.T.) ;
#19724=EDGE_CURVE('',#15147,#15191,#8239,.T.) ;
#19725=EDGE_CURVE('',#15191,#15192,#12439,.T.) ;
#19726=EDGE_CURVE('',#15192,#15174,#8240,.T.) ;
#19727=EDGE_CURVE('',#15193,#15192,#12440,.T.) ;
#19728=EDGE_CURVE('',#15194,#15193,#8241,.T.) ;
#19729=EDGE_CURVE('',#15195,#15194,#8242,.T.) ;
#19730=EDGE_CURVE('',#15195,#15196,#8243,.T.) ;
#19731=EDGE_CURVE('',#15197,#15196,#8244,.T.) ;
#19732=EDGE_CURVE('',#15198,#15197,#8245,.T.) ;
#19733=EDGE_CURVE('',#15190,#15198,#12441,.T.) ;
#19734=EDGE_CURVE('',#15191,#15184,#8246,.T.) ;
#19735=EDGE_CURVE('',#15199,#15200,#8247,.T.) ;
#19736=EDGE_CURVE('',#15201,#15199,#8248,.T.) ;
#19737=EDGE_CURVE('',#15201,#15202,#1602,.T.) ;
#19738=EDGE_CURVE('',#15202,#15203,#8249,.T.) ;
#19739=EDGE_CURVE('',#15203,#15204,#1603,.T.) ;
#19740=EDGE_CURVE('',#15200,#15204,#8250,.T.) ;
#19741=EDGE_CURVE('',#15205,#15206,#8251,.T.) ;
#19742=EDGE_CURVE('',#15207,#15205,#8252,.T.) ;
#19743=EDGE_CURVE('',#15208,#15207,#8253,.T.) ;
#19744=EDGE_CURVE('',#15206,#15208,#8254,.T.) ;
#19745=EDGE_CURVE('',#15209,#15210,#8255,.T.) ;
#19746=EDGE_CURVE('',#15211,#15209,#8256,.T.) ;
#19747=EDGE_CURVE('',#15212,#15211,#12442,.T.) ;
#19748=EDGE_CURVE('',#15213,#15212,#8257,.T.) ;
#19749=EDGE_CURVE('',#15214,#15213,#8258,.T.) ;
#19750=EDGE_CURVE('',#15215,#15214,#8259,.T.) ;
#19751=EDGE_CURVE('',#15216,#15215,#8260,.T.) ;
#19752=EDGE_CURVE('',#15217,#15216,#8261,.T.) ;
#19753=EDGE_CURVE('',#15218,#15217,#12443,.T.) ;
#19754=EDGE_CURVE('',#15210,#15218,#8262,.T.) ;
#19755=EDGE_CURVE('',#15219,#15220,#8263,.T.) ;
#19756=EDGE_CURVE('',#15219,#15221,#8264,.T.) ;
#19757=EDGE_CURVE('',#15222,#15221,#8265,.T.) ;
#19758=EDGE_CURVE('',#15220,#15222,#8266,.T.) ;
#19759=EDGE_CURVE('',#15125,#15138,#1604,.T.) ;
#19760=EDGE_CURVE('',#15137,#15126,#1605,.T.) ;
#19761=EDGE_CURVE('',#15215,#15219,#12444,.T.) ;
#19762=EDGE_CURVE('',#15221,#15214,#12445,.T.) ;
#19763=EDGE_CURVE('',#15220,#15195,#12446,.T.) ;
#19764=EDGE_CURVE('',#15196,#15222,#12447,.T.) ;
#19765=EDGE_CURVE('',#15223,#15203,#1606,.T.) ;
#19766=EDGE_CURVE('',#15202,#15224,#1607,.T.) ;
#19767=EDGE_CURVE('',#15223,#15224,#8267,.T.) ;
#19768=EDGE_CURVE('',#15186,#15225,#1608,.T.) ;
#19769=EDGE_CURVE('',#15225,#15226,#8268,.T.) ;
#19770=EDGE_CURVE('',#15226,#15187,#1609,.T.) ;
#19771=EDGE_CURVE('',#15227,#15228,#8269,.T.) ;
#19772=EDGE_CURVE('',#15229,#15227,#8270,.T.) ;
#19773=EDGE_CURVE('',#15230,#15229,#8271,.T.) ;
#19774=EDGE_CURVE('',#15228,#15230,#8272,.T.) ;
#19775=EDGE_CURVE('',#15200,#15227,#12448,.T.) ;
#19776=EDGE_CURVE('',#15229,#15204,#12449,.T.) ;
#19777=EDGE_CURVE('',#15231,#15232,#8273,.T.) ;
#19778=EDGE_CURVE('',#15233,#15231,#8274,.T.) ;
#19779=EDGE_CURVE('',#15234,#15233,#12450,.T.) ;
#19780=EDGE_CURVE('',#15235,#15234,#8275,.T.) ;
#19781=EDGE_CURVE('',#15236,#15235,#12451,.T.) ;
#19782=EDGE_CURVE('',#15232,#15236,#8276,.T.) ;
#19783=EDGE_CURVE('',#15237,#15238,#8277,.T.) ;
#19784=EDGE_CURVE('',#15239,#15237,#12452,.T.) ;
#19785=EDGE_CURVE('',#15240,#15239,#8278,.T.) ;
#19786=EDGE_CURVE('',#15241,#15240,#12453,.T.) ;
#19787=EDGE_CURVE('',#15242,#15241,#8279,.T.) ;
#19788=EDGE_CURVE('',#15238,#15242,#8280,.T.) ;
#19789=EDGE_CURVE('',#15243,#15199,#12454,.T.) ;
#19790=EDGE_CURVE('',#15243,#15244,#8281,.T.) ;
#19791=EDGE_CURVE('',#15201,#15244,#12455,.T.) ;
#19792=EDGE_CURVE('',#15245,#15243,#8282,.T.) ;
#19793=EDGE_CURVE('',#15246,#15245,#8283,.T.) ;
#19794=EDGE_CURVE('',#15244,#15246,#8284,.T.) ;
#19795=EDGE_CURVE('',#15247,#15188,#12456,.T.) ;
#19796=EDGE_CURVE('',#15247,#15225,#12457,.T.) ;
#19797=EDGE_CURVE('',#15226,#15248,#12458,.T.) ;
#19798=EDGE_CURVE('',#15184,#15248,#12459,.T.) ;
#19799=EDGE_CURVE('',#15223,#15249,#12460,.T.) ;
#19800=EDGE_CURVE('',#15229,#15249,#12461,.T.) ;
#19801=EDGE_CURVE('',#15243,#15206,#12462,.T.) ;
#19802=EDGE_CURVE('',#15206,#15199,#12463,.T.) ;
#19803=EDGE_CURVE('',#15250,#15244,#12464,.T.) ;
#19804=EDGE_CURVE('',#15250,#15224,#12465,.T.) ;
#19805=EDGE_CURVE('',#15200,#15205,#12466,.T.) ;
#19806=EDGE_CURVE('',#15205,#15227,#12467,.T.) ;
#19807=EDGE_CURVE('',#15189,#15251,#12468,.F.) ;
#19808=EDGE_CURVE('',#15251,#15247,#8285,.T.) ;
#19809=EDGE_CURVE('',#15248,#15252,#8286,.T.) ;
#19810=EDGE_CURVE('',#15252,#15191,#12469,.F.) ;
#19811=EDGE_CURVE('',#15197,#15253,#12470,.F.) ;
#19812=EDGE_CURVE('',#15253,#15251,#8287,.T.) ;
#19813=EDGE_CURVE('',#15251,#15198,#12471,.T.) ;
#19814=EDGE_CURVE('',#15193,#15252,#12472,.T.) ;
#19815=EDGE_CURVE('',#15252,#15254,#8288,.T.) ;
#19816=EDGE_CURVE('',#15254,#15194,#12473,.F.) ;
#19817=EDGE_CURVE('',#15213,#15232,#12474,.F.) ;
#19818=EDGE_CURVE('',#15214,#15236,#12475,.T.) ;
#19819=EDGE_CURVE('',#15221,#15235,#12476,.T.) ;
#19820=EDGE_CURVE('',#15222,#15234,#12477,.T.) ;
#19821=EDGE_CURVE('',#15196,#15233,#12478,.T.) ;
#19822=EDGE_CURVE('',#15231,#15197,#12479,.F.) ;
#19823=EDGE_CURVE('',#15232,#15255,#12480,.F.) ;
#19824=EDGE_CURVE('',#15255,#15253,#8289,.T.) ;
#19825=EDGE_CURVE('',#15253,#15231,#12481,.F.) ;
#19826=EDGE_CURVE('',#15242,#15254,#12482,.F.) ;
#19827=EDGE_CURVE('',#15254,#15256,#8290,.T.) ;
#19828=EDGE_CURVE('',#15256,#15238,#12483,.F.) ;
#19829=EDGE_CURVE('',#15194,#15242,#12484,.F.) ;
#19830=EDGE_CURVE('',#15195,#15241,#12485,.T.) ;
#19831=EDGE_CURVE('',#15220,#15240,#12486,.T.) ;
#19832=EDGE_CURVE('',#15219,#15239,#12487,.T.) ;
#19833=EDGE_CURVE('',#15215,#15237,#12488,.T.) ;
#19834=EDGE_CURVE('',#15238,#15216,#12489,.F.) ;
#19835=EDGE_CURVE('',#15249,#15257,#8291,.T.) ;
#19836=EDGE_CURVE('',#15257,#15230,#12490,.F.) ;
#19837=EDGE_CURVE('',#15209,#15228,#12491,.F.) ;
#19838=EDGE_CURVE('',#15230,#15211,#12492,.T.) ;
#19839=EDGE_CURVE('',#15228,#15207,#12493,.F.) ;
#19840=EDGE_CURVE('',#15208,#15245,#12494,.F.) ;
#19841=EDGE_CURVE('',#15218,#15246,#12495,.T.) ;
#19842=EDGE_CURVE('',#15245,#15210,#12496,.F.) ;
#19843=EDGE_CURVE('',#15207,#15209,#12497,.F.) ;
#19844=EDGE_CURVE('',#15210,#15208,#12498,.F.) ;
#19845=EDGE_CURVE('',#15246,#15258,#12499,.F.) ;
#19846=EDGE_CURVE('',#15258,#15250,#8292,.T.) ;
#19847=EDGE_CURVE('',#15216,#15256,#12500,.F.) ;
#19848=EDGE_CURVE('',#15256,#15258,#8293,.T.) ;
#19849=EDGE_CURVE('',#15258,#15217,#12501,.T.) ;
#19850=EDGE_CURVE('',#15212,#15257,#12502,.T.) ;
#19851=EDGE_CURVE('',#15257,#15255,#8294,.T.) ;
#19852=EDGE_CURVE('',#15255,#15213,#12503,.F.) ;
#19853=EDGE_CURVE('',#15259,#15259,#12504,.T.) ;
#19854=EDGE_CURVE('',#15259,#15260,#12505,.T.) ;
#19855=EDGE_CURVE('',#15260,#15260,#12506,.T.) ;
#19856=EDGE_CURVE('',#15261,#15261,#12507,.T.) ;
#19857=EDGE_CURVE('',#15262,#15263,#12508,.T.) ;
#19858=EDGE_CURVE('',#15263,#15262,#12509,.T.) ;
#19859=EDGE_CURVE('',#15263,#15260,#8295,.T.) ;
#19860=EDGE_CURVE('',#15261,#15262,#12510,.T.) ;
#19861=EDGE_CURVE('',#15145,#15134,#1610,.T.) ;
#19862=EDGE_CURVE('',#15133,#15146,#1611,.T.) ;
#28422=ORIENTED_EDGE('',*,*,#19617,.T.) ;
#28423=ORIENTED_EDGE('',*,*,#19618,.T.) ;
#28424=ORIENTED_EDGE('',*,*,#19619,.F.) ;
#28425=ORIENTED_EDGE('',*,*,#19620,.F.) ;
#28426=ORIENTED_EDGE('',*,*,#19621,.T.) ;
#28427=ORIENTED_EDGE('',*,*,#19622,.T.) ;
#28428=ORIENTED_EDGE('',*,*,#19617,.F.) ;
#28429=ORIENTED_EDGE('',*,*,#19623,.F.) ;
#28430=ORIENTED_EDGE('',*,*,#19624,.T.) ;
#28431=ORIENTED_EDGE('',*,*,#19625,.T.) ;
#28432=ORIENTED_EDGE('',*,*,#19621,.F.) ;
#28433=ORIENTED_EDGE('',*,*,#19626,.F.) ;
#28434=ORIENTED_EDGE('',*,*,#19627,.F.) ;
#28435=ORIENTED_EDGE('',*,*,#19628,.F.) ;
#28436=ORIENTED_EDGE('',*,*,#19629,.F.) ;
#28437=ORIENTED_EDGE('',*,*,#19630,.T.) ;
#28438=ORIENTED_EDGE('',*,*,#19631,.T.) ;
#28439=ORIENTED_EDGE('',*,*,#19632,.T.) ;
#28440=ORIENTED_EDGE('',*,*,#19633,.F.) ;
#28441=ORIENTED_EDGE('',*,*,#19634,.T.) ;
#28442=ORIENTED_EDGE('',*,*,#19635,.T.) ;
#28443=ORIENTED_EDGE('',*,*,#19636,.T.) ;
#28444=ORIENTED_EDGE('',*,*,#19631,.F.) ;
#28445=ORIENTED_EDGE('',*,*,#19637,.T.) ;
#28446=ORIENTED_EDGE('',*,*,#19638,.T.) ;
#28447=ORIENTED_EDGE('',*,*,#19639,.T.) ;
#28448=ORIENTED_EDGE('',*,*,#19635,.F.) ;
#28449=ORIENTED_EDGE('',*,*,#19640,.T.) ;
#28450=ORIENTED_EDGE('',*,*,#19641,.F.) ;
#28451=ORIENTED_EDGE('',*,*,#19642,.T.) ;
#28452=ORIENTED_EDGE('',*,*,#19643,.F.) ;
#28453=ORIENTED_EDGE('',*,*,#19644,.T.) ;
#28454=ORIENTED_EDGE('',*,*,#19641,.T.) ;
#28455=ORIENTED_EDGE('',*,*,#19645,.T.) ;
#28456=ORIENTED_EDGE('',*,*,#19638,.F.) ;
#28457=ORIENTED_EDGE('',*,*,#19646,.T.) ;
#28458=ORIENTED_EDGE('',*,*,#19627,.T.) ;
#28459=ORIENTED_EDGE('',*,*,#19647,.T.) ;
#28460=ORIENTED_EDGE('',*,*,#19624,.F.) ;
#28461=ORIENTED_EDGE('',*,*,#19648,.F.) ;
#28462=ORIENTED_EDGE('',*,*,#19649,.T.) ;
#28463=ORIENTED_EDGE('',*,*,#19650,.T.) ;
#28464=ORIENTED_EDGE('',*,*,#19651,.T.) ;
#28465=ORIENTED_EDGE('',*,*,#19652,.T.) ;
#28466=ORIENTED_EDGE('',*,*,#19653,.F.) ;
#28467=ORIENTED_EDGE('',*,*,#19654,.F.) ;
#28468=ORIENTED_EDGE('',*,*,#19655,.T.) ;
#28469=ORIENTED_EDGE('',*,*,#19656,.F.) ;
#28470=ORIENTED_EDGE('',*,*,#19657,.T.) ;
#28471=ORIENTED_EDGE('',*,*,#19658,.T.) ;
#28472=ORIENTED_EDGE('',*,*,#19654,.T.) ;
#28473=ORIENTED_EDGE('',*,*,#19659,.T.) ;
#28474=ORIENTED_EDGE('',*,*,#19660,.F.) ;
#28475=ORIENTED_EDGE('',*,*,#19661,.F.) ;
#28476=ORIENTED_EDGE('',*,*,#19662,.T.) ;
#28477=ORIENTED_EDGE('',*,*,#19663,.F.) ;
#28478=ORIENTED_EDGE('',*,*,#19664,.F.) ;
#28479=ORIENTED_EDGE('',*,*,#19665,.F.) ;
#28480=ORIENTED_EDGE('',*,*,#19666,.T.) ;
#28481=ORIENTED_EDGE('',*,*,#19667,.F.) ;
#28482=ORIENTED_EDGE('',*,*,#19668,.T.) ;
#28483=ORIENTED_EDGE('',*,*,#19669,.T.) ;
#28484=ORIENTED_EDGE('',*,*,#19665,.T.) ;
#28485=ORIENTED_EDGE('',*,*,#19670,.T.) ;
#28486=ORIENTED_EDGE('',*,*,#19671,.T.) ;
#28487=ORIENTED_EDGE('',*,*,#19672,.T.) ;
#28488=ORIENTED_EDGE('',*,*,#19668,.F.) ;
#28489=ORIENTED_EDGE('',*,*,#19673,.T.) ;
#28490=ORIENTED_EDGE('',*,*,#19656,.T.) ;
#28491=ORIENTED_EDGE('',*,*,#19674,.T.) ;
#28492=ORIENTED_EDGE('',*,*,#19671,.F.) ;
#28493=ORIENTED_EDGE('',*,*,#19675,.T.) ;
#28494=ORIENTED_EDGE('',*,*,#19676,.T.) ;
#28495=ORIENTED_EDGE('',*,*,#19677,.T.) ;
#28496=ORIENTED_EDGE('',*,*,#19667,.T.) ;
#28497=ORIENTED_EDGE('',*,*,#19678,.T.) ;
#28498=ORIENTED_EDGE('',*,*,#19679,.F.) ;
#28499=ORIENTED_EDGE('',*,*,#19680,.F.) ;
#28500=ORIENTED_EDGE('',*,*,#19681,.T.) ;
#28501=ORIENTED_EDGE('',*,*,#19682,.F.) ;
#28502=ORIENTED_EDGE('',*,*,#19683,.T.) ;
#28503=ORIENTED_EDGE('',*,*,#19684,.T.) ;
#28504=ORIENTED_EDGE('',*,*,#19680,.T.) ;
#28505=ORIENTED_EDGE('',*,*,#19685,.T.) ;
#28506=ORIENTED_EDGE('',*,*,#19686,.T.) ;
#28507=ORIENTED_EDGE('',*,*,#19687,.T.) ;
#28508=ORIENTED_EDGE('',*,*,#19661,.T.) ;
#28509=ORIENTED_EDGE('',*,*,#19688,.T.) ;
#28510=ORIENTED_EDGE('',*,*,#19689,.T.) ;
#28511=ORIENTED_EDGE('',*,*,#19690,.T.) ;
#28512=ORIENTED_EDGE('',*,*,#19686,.F.) ;
#28513=ORIENTED_EDGE('',*,*,#19691,.T.) ;
#28514=ORIENTED_EDGE('',*,*,#19682,.T.) ;
#28515=ORIENTED_EDGE('',*,*,#19692,.T.) ;
#28516=ORIENTED_EDGE('',*,*,#19689,.F.) ;
#28517=ORIENTED_EDGE('',*,*,#19693,.T.) ;
#28518=ORIENTED_EDGE('',*,*,#19679,.T.) ;
#28519=ORIENTED_EDGE('',*,*,#19694,.T.) ;
#28520=ORIENTED_EDGE('',*,*,#19664,.T.) ;
#28521=ORIENTED_EDGE('',*,*,#19695,.T.) ;
#28522=ORIENTED_EDGE('',*,*,#19696,.T.) ;
#28523=ORIENTED_EDGE('',*,*,#19697,.T.) ;
#28524=ORIENTED_EDGE('',*,*,#19663,.T.) ;
#28525=ORIENTED_EDGE('',*,*,#19698,.T.) ;
#28526=ORIENTED_EDGE('',*,*,#19653,.T.) ;
#28527=ORIENTED_EDGE('',*,*,#19699,.T.) ;
#28528=ORIENTED_EDGE('',*,*,#19660,.T.) ;
#28529=ORIENTED_EDGE('',*,*,#19700,.T.) ;
#28530=ORIENTED_EDGE('',*,*,#19683,.F.) ;
#28531=ORIENTED_EDGE('',*,*,#19649,.F.) ;
#28532=ORIENTED_EDGE('',*,*,#19701,.T.) ;
#28533=ORIENTED_EDGE('',*,*,#19651,.F.) ;
#28534=ORIENTED_EDGE('',*,*,#19676,.F.) ;
#28535=ORIENTED_EDGE('',*,*,#19702,.T.) ;
#28536=ORIENTED_EDGE('',*,*,#19703,.T.) ;
#28537=ORIENTED_EDGE('',*,*,#19704,.T.) ;
#28538=ORIENTED_EDGE('',*,*,#19705,.T.) ;
#28539=ORIENTED_EDGE('',*,*,#19706,.T.) ;
#28540=ORIENTED_EDGE('',*,*,#19703,.F.) ;
#28541=ORIENTED_EDGE('',*,*,#19696,.F.) ;
#28542=ORIENTED_EDGE('',*,*,#19707,.T.) ;
#28543=ORIENTED_EDGE('',*,*,#19657,.F.) ;
#28544=ORIENTED_EDGE('',*,*,#19705,.F.) ;
#28545=ORIENTED_EDGE('',*,*,#19708,.T.) ;
#28546=ORIENTED_EDGE('',*,*,#19670,.F.) ;
#28547=ORIENTED_EDGE('',*,*,#19694,.F.) ;
#28548=ORIENTED_EDGE('',*,*,#19693,.F.) ;
#28549=ORIENTED_EDGE('',*,*,#19709,.T.) ;
#28550=ORIENTED_EDGE('',*,*,#19702,.F.) ;
#28551=ORIENTED_EDGE('',*,*,#19710,.T.) ;
#28552=ORIENTED_EDGE('',*,*,#19711,.F.) ;
#28553=ORIENTED_EDGE('',*,*,#19712,.F.) ;
#28554=ORIENTED_EDGE('',*,*,#19678,.F.) ;
#28555=ORIENTED_EDGE('',*,*,#19666,.F.) ;
#28556=ORIENTED_EDGE('',*,*,#19669,.F.) ;
#28557=ORIENTED_EDGE('',*,*,#19672,.F.) ;
#28558=ORIENTED_EDGE('',*,*,#19674,.F.) ;
#28559=ORIENTED_EDGE('',*,*,#19655,.F.) ;
#28560=ORIENTED_EDGE('',*,*,#19658,.F.) ;
#28561=ORIENTED_EDGE('',*,*,#19713,.F.) ;
#28562=ORIENTED_EDGE('',*,*,#19714,.T.) ;
#28563=ORIENTED_EDGE('',*,*,#19715,.F.) ;
#28564=ORIENTED_EDGE('',*,*,#19716,.T.) ;
#28565=ORIENTED_EDGE('',*,*,#19710,.F.) ;
#28566=ORIENTED_EDGE('',*,*,#19708,.F.) ;
#28567=ORIENTED_EDGE('',*,*,#19717,.T.) ;
#28568=ORIENTED_EDGE('',*,*,#19718,.F.) ;
#28569=ORIENTED_EDGE('',*,*,#19713,.T.) ;
#28570=ORIENTED_EDGE('',*,*,#19704,.F.) ;
#28571=ORIENTED_EDGE('',*,*,#19719,.F.) ;
#28572=ORIENTED_EDGE('',*,*,#19720,.F.) ;
#28573=ORIENTED_EDGE('',*,*,#19717,.F.) ;
#28574=ORIENTED_EDGE('',*,*,#19650,.F.) ;
#28575=ORIENTED_EDGE('',*,*,#19685,.F.) ;
#28576=ORIENTED_EDGE('',*,*,#19695,.F.) ;
#28577=ORIENTED_EDGE('',*,*,#19677,.F.) ;
#28578=ORIENTED_EDGE('',*,*,#19697,.F.) ;
#28579=ORIENTED_EDGE('',*,*,#19706,.F.) ;
#28580=ORIENTED_EDGE('',*,*,#19659,.F.) ;
#28581=ORIENTED_EDGE('',*,*,#19700,.F.) ;
#28582=ORIENTED_EDGE('',*,*,#19675,.F.) ;
#28583=ORIENTED_EDGE('',*,*,#19721,.F.) ;
#28584=ORIENTED_EDGE('',*,*,#19688,.F.) ;
#28585=ORIENTED_EDGE('',*,*,#19699,.F.) ;
#28586=ORIENTED_EDGE('',*,*,#19673,.F.) ;
#28587=ORIENTED_EDGE('',*,*,#19709,.F.) ;
#28588=ORIENTED_EDGE('',*,*,#19691,.F.) ;
#28589=ORIENTED_EDGE('',*,*,#19721,.T.) ;
#28590=ORIENTED_EDGE('',*,*,#19707,.F.) ;
#28591=ORIENTED_EDGE('',*,*,#19722,.T.) ;
#28592=ORIENTED_EDGE('',*,*,#19723,.T.) ;
#28593=ORIENTED_EDGE('',*,*,#19719,.T.) ;
#28594=ORIENTED_EDGE('',*,*,#19701,.F.) ;
#28595=ORIENTED_EDGE('',*,*,#19724,.T.) ;
#28596=ORIENTED_EDGE('',*,*,#19725,.T.) ;
#28597=ORIENTED_EDGE('',*,*,#19726,.T.) ;
#28598=ORIENTED_EDGE('',*,*,#19684,.F.) ;
#28599=ORIENTED_EDGE('',*,*,#19726,.F.) ;
#28600=ORIENTED_EDGE('',*,*,#19727,.F.) ;
#28601=ORIENTED_EDGE('',*,*,#19728,.F.) ;
#28602=ORIENTED_EDGE('',*,*,#19729,.F.) ;
#28603=ORIENTED_EDGE('',*,*,#19730,.T.) ;
#28604=ORIENTED_EDGE('',*,*,#19731,.F.) ;
#28605=ORIENTED_EDGE('',*,*,#19732,.F.) ;
#28606=ORIENTED_EDGE('',*,*,#19733,.F.) ;
#28607=ORIENTED_EDGE('',*,*,#19722,.F.) ;
#28608=ORIENTED_EDGE('',*,*,#19698,.F.) ;
#28609=ORIENTED_EDGE('',*,*,#19662,.F.) ;
#28610=ORIENTED_EDGE('',*,*,#19687,.F.) ;
#28611=ORIENTED_EDGE('',*,*,#19690,.F.) ;
#28612=ORIENTED_EDGE('',*,*,#19692,.F.) ;
#28613=ORIENTED_EDGE('',*,*,#19681,.F.) ;
#28614=ORIENTED_EDGE('',*,*,#19652,.F.) ;
#28615=ORIENTED_EDGE('',*,*,#19712,.T.) ;
#28616=ORIENTED_EDGE('',*,*,#19734,.F.) ;
#28617=ORIENTED_EDGE('',*,*,#19724,.F.) ;
#28618=ORIENTED_EDGE('',*,*,#19735,.F.) ;
#28619=ORIENTED_EDGE('',*,*,#19736,.F.) ;
#28620=ORIENTED_EDGE('',*,*,#19737,.T.) ;
#28621=ORIENTED_EDGE('',*,*,#19738,.T.) ;
#28622=ORIENTED_EDGE('',*,*,#19739,.T.) ;
#28623=ORIENTED_EDGE('',*,*,#19740,.F.) ;
#28624=ORIENTED_EDGE('',*,*,#19741,.F.) ;
#28625=ORIENTED_EDGE('',*,*,#19742,.F.) ;
#28626=ORIENTED_EDGE('',*,*,#19743,.F.) ;
#28627=ORIENTED_EDGE('',*,*,#19744,.F.) ;
#28628=ORIENTED_EDGE('',*,*,#19745,.F.) ;
#28629=ORIENTED_EDGE('',*,*,#19746,.F.) ;
#28630=ORIENTED_EDGE('',*,*,#19747,.F.) ;
#28631=ORIENTED_EDGE('',*,*,#19748,.F.) ;
#28632=ORIENTED_EDGE('',*,*,#19749,.F.) ;
#28633=ORIENTED_EDGE('',*,*,#19750,.F.) ;
#28634=ORIENTED_EDGE('',*,*,#19751,.F.) ;
#28635=ORIENTED_EDGE('',*,*,#19752,.F.) ;
#28636=ORIENTED_EDGE('',*,*,#19753,.F.) ;
#28637=ORIENTED_EDGE('',*,*,#19754,.F.) ;
#28638=ORIENTED_EDGE('',*,*,#19755,.F.) ;
#28639=ORIENTED_EDGE('',*,*,#19756,.T.) ;
#28640=ORIENTED_EDGE('',*,*,#19757,.F.) ;
#28641=ORIENTED_EDGE('',*,*,#19758,.F.) ;
#28642=ORIENTED_EDGE('',*,*,#19759,.T.) ;
#28643=ORIENTED_EDGE('',*,*,#19633,.T.) ;
#28644=ORIENTED_EDGE('',*,*,#19760,.T.) ;
#28645=ORIENTED_EDGE('',*,*,#19619,.T.) ;
#28646=ORIENTED_EDGE('',*,*,#19761,.F.) ;
#28647=ORIENTED_EDGE('',*,*,#19750,.T.) ;
#28648=ORIENTED_EDGE('',*,*,#19762,.F.) ;
#28649=ORIENTED_EDGE('',*,*,#19756,.F.) ;
#28650=ORIENTED_EDGE('',*,*,#19763,.F.) ;
#28651=ORIENTED_EDGE('',*,*,#19758,.T.) ;
#28652=ORIENTED_EDGE('',*,*,#19764,.F.) ;
#28653=ORIENTED_EDGE('',*,*,#19730,.F.) ;
#28654=ORIENTED_EDGE('',*,*,#19765,.T.) ;
#28655=ORIENTED_EDGE('',*,*,#19738,.F.) ;
#28656=ORIENTED_EDGE('',*,*,#19766,.T.) ;
#28657=ORIENTED_EDGE('',*,*,#19767,.F.) ;
#28658=ORIENTED_EDGE('',*,*,#19768,.T.) ;
#28659=ORIENTED_EDGE('',*,*,#19769,.T.) ;
#28660=ORIENTED_EDGE('',*,*,#19770,.T.) ;
#28661=ORIENTED_EDGE('',*,*,#19715,.T.) ;
#28662=ORIENTED_EDGE('',*,*,#19771,.F.) ;
#28663=ORIENTED_EDGE('',*,*,#19772,.F.) ;
#28664=ORIENTED_EDGE('',*,*,#19773,.F.) ;
#28665=ORIENTED_EDGE('',*,*,#19774,.F.) ;
#28666=ORIENTED_EDGE('',*,*,#19775,.F.) ;
#28667=ORIENTED_EDGE('',*,*,#19740,.T.) ;
#28668=ORIENTED_EDGE('',*,*,#19776,.F.) ;
#28669=ORIENTED_EDGE('',*,*,#19772,.T.) ;
#28670=ORIENTED_EDGE('',*,*,#19777,.F.) ;
#28671=ORIENTED_EDGE('',*,*,#19778,.F.) ;
#28672=ORIENTED_EDGE('',*,*,#19779,.F.) ;
#28673=ORIENTED_EDGE('',*,*,#19780,.F.) ;
#28674=ORIENTED_EDGE('',*,*,#19781,.F.) ;
#28675=ORIENTED_EDGE('',*,*,#19782,.F.) ;
#28676=ORIENTED_EDGE('',*,*,#19783,.F.) ;
#28677=ORIENTED_EDGE('',*,*,#19784,.F.) ;
#28678=ORIENTED_EDGE('',*,*,#19785,.F.) ;
#28679=ORIENTED_EDGE('',*,*,#19786,.F.) ;
#28680=ORIENTED_EDGE('',*,*,#19787,.F.) ;
#28681=ORIENTED_EDGE('',*,*,#19788,.F.) ;
#28682=ORIENTED_EDGE('',*,*,#19789,.F.) ;
#28683=ORIENTED_EDGE('',*,*,#19790,.T.) ;
#28684=ORIENTED_EDGE('',*,*,#19791,.F.) ;
#28685=ORIENTED_EDGE('',*,*,#19736,.T.) ;
#28686=ORIENTED_EDGE('',*,*,#19792,.F.) ;
#28687=ORIENTED_EDGE('',*,*,#19793,.F.) ;
#28688=ORIENTED_EDGE('',*,*,#19794,.F.) ;
#28689=ORIENTED_EDGE('',*,*,#19790,.F.) ;
#28690=ORIENTED_EDGE('',*,*,#19714,.F.) ;
#28691=ORIENTED_EDGE('',*,*,#19718,.T.) ;
#28692=ORIENTED_EDGE('',*,*,#19795,.F.) ;
#28693=ORIENTED_EDGE('',*,*,#19796,.T.) ;
#28694=ORIENTED_EDGE('',*,*,#19768,.F.) ;
#28695=ORIENTED_EDGE('',*,*,#19770,.F.) ;
#28696=ORIENTED_EDGE('',*,*,#19797,.T.) ;
#28697=ORIENTED_EDGE('',*,*,#19798,.F.) ;
#28698=ORIENTED_EDGE('',*,*,#19711,.T.) ;
#28699=ORIENTED_EDGE('',*,*,#19716,.F.) ;
#28700=ORIENTED_EDGE('',*,*,#19765,.F.) ;
#28701=ORIENTED_EDGE('',*,*,#19799,.T.) ;
#28702=ORIENTED_EDGE('',*,*,#19800,.F.) ;
#28703=ORIENTED_EDGE('',*,*,#19776,.T.) ;
#28704=ORIENTED_EDGE('',*,*,#19739,.F.) ;
#28705=ORIENTED_EDGE('',*,*,#19801,.F.) ;
#28706=ORIENTED_EDGE('',*,*,#19789,.T.) ;
#28707=ORIENTED_EDGE('',*,*,#19802,.F.) ;
#28708=ORIENTED_EDGE('',*,*,#19737,.F.) ;
#28709=ORIENTED_EDGE('',*,*,#19791,.T.) ;
#28710=ORIENTED_EDGE('',*,*,#19803,.F.) ;
#28711=ORIENTED_EDGE('',*,*,#19804,.T.) ;
#28712=ORIENTED_EDGE('',*,*,#19766,.F.) ;
#28713=ORIENTED_EDGE('',*,*,#19805,.F.) ;
#28714=ORIENTED_EDGE('',*,*,#19775,.T.) ;
#28715=ORIENTED_EDGE('',*,*,#19806,.F.) ;
#28716=ORIENTED_EDGE('',*,*,#19735,.T.) ;
#28717=ORIENTED_EDGE('',*,*,#19805,.T.) ;
#28718=ORIENTED_EDGE('',*,*,#19741,.T.) ;
#28719=ORIENTED_EDGE('',*,*,#19802,.T.) ;
#28720=ORIENTED_EDGE('',*,*,#19795,.T.) ;
#28721=ORIENTED_EDGE('',*,*,#19720,.T.) ;
#28722=ORIENTED_EDGE('',*,*,#19807,.T.) ;
#28723=ORIENTED_EDGE('',*,*,#19808,.T.) ;
#28724=ORIENTED_EDGE('',*,*,#19798,.T.) ;
#28725=ORIENTED_EDGE('',*,*,#19809,.T.) ;
#28726=ORIENTED_EDGE('',*,*,#19810,.T.) ;
#28727=ORIENTED_EDGE('',*,*,#19734,.T.) ;
#28728=ORIENTED_EDGE('',*,*,#19811,.T.) ;
#28729=ORIENTED_EDGE('',*,*,#19812,.T.) ;
#28730=ORIENTED_EDGE('',*,*,#19813,.T.) ;
#28731=ORIENTED_EDGE('',*,*,#19732,.T.) ;
#28732=ORIENTED_EDGE('',*,*,#19814,.T.) ;
#28733=ORIENTED_EDGE('',*,*,#19815,.T.) ;
#28734=ORIENTED_EDGE('',*,*,#19816,.T.) ;
#28735=ORIENTED_EDGE('',*,*,#19728,.T.) ;
#28736=ORIENTED_EDGE('',*,*,#19817,.T.) ;
#28737=ORIENTED_EDGE('',*,*,#19782,.T.) ;
#28738=ORIENTED_EDGE('',*,*,#19818,.F.) ;
#28739=ORIENTED_EDGE('',*,*,#19749,.T.) ;
#28740=ORIENTED_EDGE('',*,*,#19818,.T.) ;
#28741=ORIENTED_EDGE('',*,*,#19781,.T.) ;
#28742=ORIENTED_EDGE('',*,*,#19819,.F.) ;
#28743=ORIENTED_EDGE('',*,*,#19762,.T.) ;
#28744=ORIENTED_EDGE('',*,*,#19819,.T.) ;
#28745=ORIENTED_EDGE('',*,*,#19780,.T.) ;
#28746=ORIENTED_EDGE('',*,*,#19820,.F.) ;
#28747=ORIENTED_EDGE('',*,*,#19757,.T.) ;
#28748=ORIENTED_EDGE('',*,*,#19820,.T.) ;
#28749=ORIENTED_EDGE('',*,*,#19779,.T.) ;
#28750=ORIENTED_EDGE('',*,*,#19821,.F.) ;
#28751=ORIENTED_EDGE('',*,*,#19764,.T.) ;
#28752=ORIENTED_EDGE('',*,*,#19821,.T.) ;
#28753=ORIENTED_EDGE('',*,*,#19778,.T.) ;
#28754=ORIENTED_EDGE('',*,*,#19822,.T.) ;
#28755=ORIENTED_EDGE('',*,*,#19731,.T.) ;
#28756=ORIENTED_EDGE('',*,*,#19823,.T.) ;
#28757=ORIENTED_EDGE('',*,*,#19824,.T.) ;
#28758=ORIENTED_EDGE('',*,*,#19825,.T.) ;
#28759=ORIENTED_EDGE('',*,*,#19777,.T.) ;
#28760=ORIENTED_EDGE('',*,*,#19826,.T.) ;
#28761=ORIENTED_EDGE('',*,*,#19827,.T.) ;
#28762=ORIENTED_EDGE('',*,*,#19828,.T.) ;
#28763=ORIENTED_EDGE('',*,*,#19788,.T.) ;
#28764=ORIENTED_EDGE('',*,*,#19829,.T.) ;
#28765=ORIENTED_EDGE('',*,*,#19787,.T.) ;
#28766=ORIENTED_EDGE('',*,*,#19830,.F.) ;
#28767=ORIENTED_EDGE('',*,*,#19729,.T.) ;
#28768=ORIENTED_EDGE('',*,*,#19830,.T.) ;
#28769=ORIENTED_EDGE('',*,*,#19786,.T.) ;
#28770=ORIENTED_EDGE('',*,*,#19831,.F.) ;
#28771=ORIENTED_EDGE('',*,*,#19763,.T.) ;
#28772=ORIENTED_EDGE('',*,*,#19831,.T.) ;
#28773=ORIENTED_EDGE('',*,*,#19785,.T.) ;
#28774=ORIENTED_EDGE('',*,*,#19832,.F.) ;
#28775=ORIENTED_EDGE('',*,*,#19755,.T.) ;
#28776=ORIENTED_EDGE('',*,*,#19832,.T.) ;
#28777=ORIENTED_EDGE('',*,*,#19784,.T.) ;
#28778=ORIENTED_EDGE('',*,*,#19833,.F.) ;
#28779=ORIENTED_EDGE('',*,*,#19761,.T.) ;
#28780=ORIENTED_EDGE('',*,*,#19833,.T.) ;
#28781=ORIENTED_EDGE('',*,*,#19783,.T.) ;
#28782=ORIENTED_EDGE('',*,*,#19834,.T.) ;
#28783=ORIENTED_EDGE('',*,*,#19751,.T.) ;
#28784=ORIENTED_EDGE('',*,*,#19800,.T.) ;
#28785=ORIENTED_EDGE('',*,*,#19835,.T.) ;
#28786=ORIENTED_EDGE('',*,*,#19836,.T.) ;
#28787=ORIENTED_EDGE('',*,*,#19773,.T.) ;
#28788=ORIENTED_EDGE('',*,*,#19837,.T.) ;
#28789=ORIENTED_EDGE('',*,*,#19774,.T.) ;
#28790=ORIENTED_EDGE('',*,*,#19838,.T.) ;
#28791=ORIENTED_EDGE('',*,*,#19746,.T.) ;
#28792=ORIENTED_EDGE('',*,*,#19806,.T.) ;
#28793=ORIENTED_EDGE('',*,*,#19771,.T.) ;
#28794=ORIENTED_EDGE('',*,*,#19839,.T.) ;
#28795=ORIENTED_EDGE('',*,*,#19742,.T.) ;
#28796=ORIENTED_EDGE('',*,*,#19801,.T.) ;
#28797=ORIENTED_EDGE('',*,*,#19744,.T.) ;
#28798=ORIENTED_EDGE('',*,*,#19840,.T.) ;
#28799=ORIENTED_EDGE('',*,*,#19792,.T.) ;
#28800=ORIENTED_EDGE('',*,*,#19841,.T.) ;
#28801=ORIENTED_EDGE('',*,*,#19793,.T.) ;
#28802=ORIENTED_EDGE('',*,*,#19842,.T.) ;
#28803=ORIENTED_EDGE('',*,*,#19754,.T.) ;
#28804=ORIENTED_EDGE('',*,*,#19743,.T.) ;
#28805=ORIENTED_EDGE('',*,*,#19843,.T.) ;
#28806=ORIENTED_EDGE('',*,*,#19745,.T.) ;
#28807=ORIENTED_EDGE('',*,*,#19844,.T.) ;
#28808=ORIENTED_EDGE('',*,*,#19840,.F.) ;
#28809=ORIENTED_EDGE('',*,*,#19844,.F.) ;
#28810=ORIENTED_EDGE('',*,*,#19842,.F.) ;
#28811=ORIENTED_EDGE('',*,*,#19837,.F.) ;
#28812=ORIENTED_EDGE('',*,*,#19843,.F.) ;
#28813=ORIENTED_EDGE('',*,*,#19839,.F.) ;
#28814=ORIENTED_EDGE('',*,*,#19803,.T.) ;
#28815=ORIENTED_EDGE('',*,*,#19794,.T.) ;
#28816=ORIENTED_EDGE('',*,*,#19845,.T.) ;
#28817=ORIENTED_EDGE('',*,*,#19846,.T.) ;
#28818=ORIENTED_EDGE('',*,*,#19847,.T.) ;
#28819=ORIENTED_EDGE('',*,*,#19848,.T.) ;
#28820=ORIENTED_EDGE('',*,*,#19849,.T.) ;
#28821=ORIENTED_EDGE('',*,*,#19752,.T.) ;
#28822=ORIENTED_EDGE('',*,*,#19753,.T.) ;
#28823=ORIENTED_EDGE('',*,*,#19849,.F.) ;
#28824=ORIENTED_EDGE('',*,*,#19845,.F.) ;
#28825=ORIENTED_EDGE('',*,*,#19841,.F.) ;
#28826=ORIENTED_EDGE('',*,*,#19850,.T.) ;
#28827=ORIENTED_EDGE('',*,*,#19851,.T.) ;
#28828=ORIENTED_EDGE('',*,*,#19852,.T.) ;
#28829=ORIENTED_EDGE('',*,*,#19748,.T.) ;
#28830=ORIENTED_EDGE('',*,*,#19836,.F.) ;
#28831=ORIENTED_EDGE('',*,*,#19850,.F.) ;
#28832=ORIENTED_EDGE('',*,*,#19747,.T.) ;
#28833=ORIENTED_EDGE('',*,*,#19838,.F.) ;
#28834=ORIENTED_EDGE('',*,*,#19828,.F.) ;
#28835=ORIENTED_EDGE('',*,*,#19847,.F.) ;
#28836=ORIENTED_EDGE('',*,*,#19834,.F.) ;
#28837=ORIENTED_EDGE('',*,*,#19817,.F.) ;
#28838=ORIENTED_EDGE('',*,*,#19852,.F.) ;
#28839=ORIENTED_EDGE('',*,*,#19823,.F.) ;
#28840=ORIENTED_EDGE('',*,*,#19816,.F.) ;
#28841=ORIENTED_EDGE('',*,*,#19826,.F.) ;
#28842=ORIENTED_EDGE('',*,*,#19829,.F.) ;
#28843=ORIENTED_EDGE('',*,*,#19822,.F.) ;
#28844=ORIENTED_EDGE('',*,*,#19825,.F.) ;
#28845=ORIENTED_EDGE('',*,*,#19811,.F.) ;
#28846=ORIENTED_EDGE('',*,*,#19810,.F.) ;
#28847=ORIENTED_EDGE('',*,*,#19814,.F.) ;
#28848=ORIENTED_EDGE('',*,*,#19727,.T.) ;
#28849=ORIENTED_EDGE('',*,*,#19725,.F.) ;
#28850=ORIENTED_EDGE('',*,*,#19733,.T.) ;
#28851=ORIENTED_EDGE('',*,*,#19813,.F.) ;
#28852=ORIENTED_EDGE('',*,*,#19807,.F.) ;
#28853=ORIENTED_EDGE('',*,*,#19723,.F.) ;
#28854=ORIENTED_EDGE('',*,*,#19853,.T.) ;
#28855=ORIENTED_EDGE('',*,*,#19854,.T.) ;
#28856=ORIENTED_EDGE('',*,*,#19855,.T.) ;
#28857=ORIENTED_EDGE('',*,*,#19854,.F.) ;
#28858=ORIENTED_EDGE('',*,*,#19799,.F.) ;
#28859=ORIENTED_EDGE('',*,*,#19767,.T.) ;
#28860=ORIENTED_EDGE('',*,*,#19804,.F.) ;
#28861=ORIENTED_EDGE('',*,*,#19846,.F.) ;
#28862=ORIENTED_EDGE('',*,*,#19848,.F.) ;
#28863=ORIENTED_EDGE('',*,*,#19827,.F.) ;
#28864=ORIENTED_EDGE('',*,*,#19815,.F.) ;
#28865=ORIENTED_EDGE('',*,*,#19809,.F.) ;
#28866=ORIENTED_EDGE('',*,*,#19797,.F.) ;
#28867=ORIENTED_EDGE('',*,*,#19769,.F.) ;
#28868=ORIENTED_EDGE('',*,*,#19796,.F.) ;
#28869=ORIENTED_EDGE('',*,*,#19808,.F.) ;
#28870=ORIENTED_EDGE('',*,*,#19812,.F.) ;
#28871=ORIENTED_EDGE('',*,*,#19824,.F.) ;
#28872=ORIENTED_EDGE('',*,*,#19851,.F.) ;
#28873=ORIENTED_EDGE('',*,*,#19835,.F.) ;
#28874=ORIENTED_EDGE('',*,*,#19856,.F.) ;
#28875=ORIENTED_EDGE('',*,*,#19857,.F.) ;
#28876=ORIENTED_EDGE('',*,*,#19858,.F.) ;
#28877=ORIENTED_EDGE('',*,*,#19859,.T.) ;
#28878=ORIENTED_EDGE('',*,*,#19855,.F.) ;
#28879=ORIENTED_EDGE('',*,*,#19859,.F.) ;
#28880=ORIENTED_EDGE('',*,*,#19856,.T.) ;
#28881=ORIENTED_EDGE('',*,*,#19860,.T.) ;
#28882=ORIENTED_EDGE('',*,*,#19857,.T.) ;
#28883=ORIENTED_EDGE('',*,*,#19858,.T.) ;
#28884=ORIENTED_EDGE('',*,*,#19860,.F.) ;
#28885=ORIENTED_EDGE('',*,*,#19853,.F.) ;
#28886=ORIENTED_EDGE('',*,*,#19861,.T.) ;
#28887=ORIENTED_EDGE('',*,*,#19629,.T.) ;
#28888=ORIENTED_EDGE('',*,*,#19862,.T.) ;
#28889=ORIENTED_EDGE('',*,*,#19643,.T.) ;
#28890=ORIENTED_EDGE('',*,*,#19760,.F.) ;
#28891=ORIENTED_EDGE('',*,*,#19632,.F.) ;
#28892=ORIENTED_EDGE('',*,*,#19636,.F.) ;
#28893=ORIENTED_EDGE('',*,*,#19639,.F.) ;
#28894=ORIENTED_EDGE('',*,*,#19645,.F.) ;
#28895=ORIENTED_EDGE('',*,*,#19644,.F.) ;
#28896=ORIENTED_EDGE('',*,*,#19862,.F.) ;
#28897=ORIENTED_EDGE('',*,*,#19628,.T.) ;
#28898=ORIENTED_EDGE('',*,*,#19648,.T.) ;
#28899=ORIENTED_EDGE('',*,*,#19626,.T.) ;
#28900=ORIENTED_EDGE('',*,*,#19623,.T.) ;
#28901=ORIENTED_EDGE('',*,*,#19620,.T.) ;
#28902=ORIENTED_EDGE('',*,*,#19759,.F.) ;
#28903=ORIENTED_EDGE('',*,*,#19618,.F.) ;
#28904=ORIENTED_EDGE('',*,*,#19622,.F.) ;
#28905=ORIENTED_EDGE('',*,*,#19625,.F.) ;
#28906=ORIENTED_EDGE('',*,*,#19647,.F.) ;
#28907=ORIENTED_EDGE('',*,*,#19630,.F.) ;
#28908=ORIENTED_EDGE('',*,*,#19861,.F.) ;
#28909=ORIENTED_EDGE('',*,*,#19642,.F.) ;
#28910=ORIENTED_EDGE('',*,*,#19646,.F.) ;
#28911=ORIENTED_EDGE('',*,*,#19640,.F.) ;
#28912=ORIENTED_EDGE('',*,*,#19637,.F.) ;
#28913=ORIENTED_EDGE('',*,*,#19634,.F.) ;
#30614=CYLINDRICAL_SURFACE('',#35913,1.7526) ;
#30615=CYLINDRICAL_SURFACE('',#35915,1.7526) ;
#30616=CYLINDRICAL_SURFACE('',#35916,1.7526) ;
#30617=CYLINDRICAL_SURFACE('',#35917,1.7526) ;
#30618=CYLINDRICAL_SURFACE('',#35919,1.5) ;
#30619=CYLINDRICAL_SURFACE('',#35921,1.5) ;
#30620=CYLINDRICAL_SURFACE('',#35922,1.5) ;
#30621=CYLINDRICAL_SURFACE('',#35923,1.5) ;
#30622=CYLINDRICAL_SURFACE('',#35925,1.5) ;
#30623=CYLINDRICAL_SURFACE('',#35926,1.7526) ;
#30624=CYLINDRICAL_SURFACE('',#35927,0.125) ;
#30625=CYLINDRICAL_SURFACE('',#35935,0.125) ;
#30626=CYLINDRICAL_SURFACE('',#35947,0.125) ;
#30627=CYLINDRICAL_SURFACE('',#35953,0.125) ;
#30628=CYLINDRICAL_SURFACE('',#35954,0.125) ;
#30629=CYLINDRICAL_SURFACE('',#35961,0.125) ;
#30630=CYLINDRICAL_SURFACE('',#35963,0.125) ;
#30631=CYLINDRICAL_SURFACE('',#35969,0.125) ;
#30632=CYLINDRICAL_SURFACE('',#35970,0.0635000000000012) ;
#30633=CYLINDRICAL_SURFACE('',#35971,0.125) ;
#30634=CYLINDRICAL_SURFACE('',#35973,0.0634999999999974) ;
#30635=CYLINDRICAL_SURFACE('',#35978,0.125) ;
#30636=CYLINDRICAL_SURFACE('',#35986,0.125) ;
#30637=CYLINDRICAL_SURFACE('',#35989,0.125) ;
#30638=CYLINDRICAL_SURFACE('',#35995,0.634999999999996) ;
#30639=CYLINDRICAL_SURFACE('',#35996,0.125) ;
#30640=CYLINDRICAL_SURFACE('',#35998,0.125) ;
#30641=CYLINDRICAL_SURFACE('',#36010,0.698499999999999) ;
#30642=CYLINDRICAL_SURFACE('',#36013,0.698500000000001) ;
#30643=CYLINDRICAL_SURFACE('',#36016,0.0634999999999973) ;
#30644=CYLINDRICAL_SURFACE('',#36017,0.0635000000000008) ;
#30645=CYLINDRICAL_SURFACE('',#36019,0.125) ;
#30646=CYLINDRICAL_SURFACE('',#36028,0.125) ;
#30647=CYLINDRICAL_SURFACE('',#36050,0.125) ;
#30648=CYLINDRICAL_SURFACE('',#36051,0.125) ;
#30649=CYLINDRICAL_SURFACE('',#36053,0.125) ;
#30650=CYLINDRICAL_SURFACE('',#36055,0.125) ;
#30651=CYLINDRICAL_SURFACE('',#36058,0.125) ;
#30652=CYLINDRICAL_SURFACE('',#36061,0.125) ;
#30653=CYLINDRICAL_SURFACE('',#36066,0.125) ;
#30654=CYLINDRICAL_SURFACE('',#36070,0.125) ;
#30655=CYLINDRICAL_SURFACE('',#36072,0.125) ;
#30656=CYLINDRICAL_SURFACE('',#36075,0.125) ;
#30657=CYLINDRICAL_SURFACE('',#36078,0.125) ;
#30658=CYLINDRICAL_SURFACE('',#36083,0.125) ;
#30659=CYLINDRICAL_SURFACE('',#36087,0.125) ;
#30660=CYLINDRICAL_SURFACE('',#36089,0.125) ;
#30661=CYLINDRICAL_SURFACE('',#36091,0.125) ;
#30662=CYLINDRICAL_SURFACE('',#36094,0.125) ;
#30663=CYLINDRICAL_SURFACE('',#36096,0.125) ;
#30664=CYLINDRICAL_SURFACE('',#36098,0.125) ;
#30665=CYLINDRICAL_SURFACE('',#36101,0.125) ;
#30666=CYLINDRICAL_SURFACE('',#36106,0.125) ;
#30667=CYLINDRICAL_SURFACE('',#36108,0.125) ;
#30668=CYLINDRICAL_SURFACE('',#36112,0.125) ;
#30669=CYLINDRICAL_SURFACE('',#36128,2.8575) ;
#32332=ADVANCED_FACE('',(#3853),#30614,.F.) ;
#32333=ADVANCED_FACE('',(#3854),#30615,.F.) ;
#32334=ADVANCED_FACE('',(#3855),#30616,.F.) ;
#32335=ADVANCED_FACE('',(#3856),#30617,.F.) ;
#32336=ADVANCED_FACE('',(#3857),#30618,.F.) ;
#32337=ADVANCED_FACE('',(#3858),#30619,.F.) ;
#32338=ADVANCED_FACE('',(#3859),#30620,.F.) ;
#32339=ADVANCED_FACE('',(#3860),#30621,.F.) ;
#32340=ADVANCED_FACE('',(#3861),#30622,.F.) ;
#32341=ADVANCED_FACE('',(#3862),#30623,.F.) ;
#32342=ADVANCED_FACE('',(#3863),#30624,.T.) ;
#32343=ADVANCED_FACE('',(#3864),#436,.T.) ;
#32344=ADVANCED_FACE('',(#3865),#30625,.T.) ;
#32345=ADVANCED_FACE('',(#3866),#437,.T.) ;
#32346=ADVANCED_FACE('',(#3867),#438,.T.) ;
#32347=ADVANCED_FACE('',(#3868),#30626,.T.) ;
#32348=ADVANCED_FACE('',(#3869),#439,.T.) ;
#32349=ADVANCED_FACE('',(#3870),#30627,.T.) ;
#32350=ADVANCED_FACE('',(#3871),#30628,.T.) ;
#32351=ADVANCED_FACE('',(#3872),#440,.T.) ;
#32352=ADVANCED_FACE('',(#3873),#30629,.T.) ;
#32353=ADVANCED_FACE('',(#3874),#30630,.T.) ;
#32354=ADVANCED_FACE('',(#3875),#441,.T.) ;
#32355=ADVANCED_FACE('',(#3876),#30631,.T.) ;
#32356=ADVANCED_FACE('',(#3877),#30632,.F.) ;
#32357=ADVANCED_FACE('',(#3878),#30633,.T.) ;
#32358=ADVANCED_FACE('',(#3879),#30634,.F.) ;
#32359=ADVANCED_FACE('',(#3880),#109,.T.) ;
#32360=ADVANCED_FACE('',(#3881),#110,.T.) ;
#32361=ADVANCED_FACE('',(#3882),#30635,.T.) ;
#32362=ADVANCED_FACE('',(#3883),#111,.T.) ;
#32363=ADVANCED_FACE('',(#3884),#112,.T.) ;
#32364=ADVANCED_FACE('',(#3885),#2173,.T.) ;
#32365=ADVANCED_FACE('',(#3886),#30636,.T.) ;
#32366=ADVANCED_FACE('',(#3887),#2174,.T.) ;
#32367=ADVANCED_FACE('',(#3888),#30637,.T.) ;
#32368=ADVANCED_FACE('',(#3889),#2175,.T.) ;
#32369=ADVANCED_FACE('',(#3890),#2176,.T.) ;
#32370=ADVANCED_FACE('',(#3891),#2177,.T.) ;
#32371=ADVANCED_FACE('',(#3892),#2178,.T.) ;
#32372=ADVANCED_FACE('',(#3893),#30638,.T.) ;
#32373=ADVANCED_FACE('',(#3894),#30639,.T.) ;
#32374=ADVANCED_FACE('',(#3895),#30640,.T.) ;
#32375=ADVANCED_FACE('',(#3896),#2179,.T.) ;
#32376=ADVANCED_FACE('',(#3897),#2180,.T.) ;
#32377=ADVANCED_FACE('',(#3898),#2181,.T.) ;
#32378=ADVANCED_FACE('',(#3899),#2182,.T.) ;
#32379=ADVANCED_FACE('',(#3900),#2183,.T.) ;
#32380=ADVANCED_FACE('',(#3901,#1170),#2184,.T.) ;
#32381=ADVANCED_FACE('',(#3902),#30641,.T.) ;
#32382=ADVANCED_FACE('',(#3903),#30642,.T.) ;
#32383=ADVANCED_FACE('',(#3904),#30643,.F.) ;
#32384=ADVANCED_FACE('',(#3905),#30644,.F.) ;
#32385=ADVANCED_FACE('',(#3906),#2185,.T.) ;
#32386=ADVANCED_FACE('',(#3907),#30645,.T.) ;
#32387=ADVANCED_FACE('',(#3908),#2186,.T.) ;
#32388=ADVANCED_FACE('',(#3909),#2187,.T.) ;
#32389=ADVANCED_FACE('',(#3910),#30646,.T.) ;
#32390=ADVANCED_FACE('',(#3911),#2188,.T.) ;
#32391=ADVANCED_FACE('',(#3912),#442,.F.) ;
#32392=ADVANCED_FACE('',(#3913),#443,.F.) ;
#32393=ADVANCED_FACE('',(#3914),#444,.F.) ;
#32394=ADVANCED_FACE('',(#3915),#113,.T.) ;
#32395=ADVANCED_FACE('',(#3916),#445,.F.) ;
#32396=ADVANCED_FACE('',(#3917),#114,.T.) ;
#32397=ADVANCED_FACE('',(#3918),#30647,.T.) ;
#32398=ADVANCED_FACE('',(#3919),#30648,.F.) ;
#32399=ADVANCED_FACE('',(#3920),#30649,.F.) ;
#32400=ADVANCED_FACE('',(#3921),#30650,.T.) ;
#32401=ADVANCED_FACE('',(#3922),#30651,.T.) ;
#32402=ADVANCED_FACE('',(#3923),#30652,.T.) ;
#32403=ADVANCED_FACE('',(#3924),#446,.T.) ;
#32404=ADVANCED_FACE('',(#3925),#30653,.T.) ;
#32405=ADVANCED_FACE('',(#3926),#447,.T.) ;
#32406=ADVANCED_FACE('',(#3927),#30654,.T.) ;
#32407=ADVANCED_FACE('',(#3928),#30655,.T.) ;
#32408=ADVANCED_FACE('',(#3929),#30656,.T.) ;
#32409=ADVANCED_FACE('',(#3930),#30657,.T.) ;
#32410=ADVANCED_FACE('',(#3931),#448,.T.) ;
#32411=ADVANCED_FACE('',(#3932),#30658,.T.) ;
#32412=ADVANCED_FACE('',(#3933),#449,.T.) ;
#32413=ADVANCED_FACE('',(#3934),#30659,.T.) ;
#32414=ADVANCED_FACE('',(#3935),#30660,.F.) ;
#32415=ADVANCED_FACE('',(#3936),#30661,.T.) ;
#32416=ADVANCED_FACE('',(#3937),#30662,.T.) ;
#32417=ADVANCED_FACE('',(#3938),#30663,.T.) ;
#32418=ADVANCED_FACE('',(#3939),#30664,.T.) ;
#32419=ADVANCED_FACE('',(#3940),#30665,.T.) ;
#32420=ADVANCED_FACE('',(#3941),#115,.T.) ;
#32421=ADVANCED_FACE('',(#3942),#116,.T.) ;
#32422=ADVANCED_FACE('',(#3943),#30666,.F.) ;
#32423=ADVANCED_FACE('',(#3944),#30667,.T.) ;
#32424=ADVANCED_FACE('',(#3945),#450,.T.) ;
#32425=ADVANCED_FACE('',(#3946),#30668,.T.) ;
#32426=ADVANCED_FACE('',(#3947),#451,.T.) ;
#32427=ADVANCED_FACE('',(#3948),#117,.T.) ;
#32428=ADVANCED_FACE('',(#3949),#118,.T.) ;
#32429=ADVANCED_FACE('',(#3950),#119,.T.) ;
#32430=ADVANCED_FACE('',(#3951),#120,.T.) ;
#32431=ADVANCED_FACE('',(#3952),#452,.T.) ;
#32432=ADVANCED_FACE('',(#3953),#453,.T.) ;
#32433=ADVANCED_FACE('',(#3954),#454,.T.) ;
#32434=ADVANCED_FACE('',(#3955,#1171),#2189,.T.) ;
#32435=ADVANCED_FACE('',(#3956),#30669,.T.) ;
#32436=ADVANCED_FACE('',(#3957),#455,.F.) ;
#32437=ADVANCED_FACE('',(#3958,#1172),#2190,.T.) ;
#32438=ADVANCED_FACE('',(#3959),#746,.F.) ;
#32439=ADVANCED_FACE('',(#3960),#747,.F.) ;
#32643=CLOSED_SHELL('',(#32332,#32333,#32334,#32335,#32336,#32337,#32338,
#32339,#32340,#32341,#32342,#32343,#32344,#32345,#32346,#32347,#32348,#32349,
#32350,#32351,#32352,#32353,#32354,#32355,#32356,#32357,#32358,#32359,#32360,
#32361,#32362,#32363,#32364,#32365,#32366,#32367,#32368,#32369,#32370,#32371,
#32372,#32373,#32374,#32375,#32376,#32377,#32378,#32379,#32380,#32381,#32382,
#32383,#32384,#32385,#32386,#32387,#32388,#32389,#32390,#32391,#32392,#32393,
#32394,#32395,#32396,#32397,#32398,#32399,#32400,#32401,#32402,#32403,#32404,
#32405,#32406,#32407,#32408,#32409,#32410,#32411,#32412,#32413,#32414,#32415,
#32416,#32417,#32418,#32419,#32420,#32421,#32422,#32423,#32424,#32425,#32426,
#32427,#32428,#32429,#32430,#32431,#32432,#32433,#32434,#32435,#32436,#32437,
#32438,#32439)) ;
#35912=AXIS2_PLACEMENT_3D('',#78787,#44767,#44768) ;
#35913=AXIS2_PLACEMENT_3D('',#78788,#44769,#44770) ;
#35914=AXIS2_PLACEMENT_3D('',#78810,#44772,#44773) ;
#35915=AXIS2_PLACEMENT_3D('',#78831,#44774,#44775) ;
#35916=AXIS2_PLACEMENT_3D('',#78907,#44777,#44778) ;
#35917=AXIS2_PLACEMENT_3D('',#78983,#44780,#44781) ;
#35918=AXIS2_PLACEMENT_3D('',#79003,#44783,#44784) ;
#35919=AXIS2_PLACEMENT_3D('',#79022,#44785,#44786) ;
#35920=AXIS2_PLACEMENT_3D('',#79038,#44788,#44789) ;
#35921=AXIS2_PLACEMENT_3D('',#79065,#44790,#44791) ;
#35922=AXIS2_PLACEMENT_3D('',#79141,#44793,#44794) ;
#35923=AXIS2_PLACEMENT_3D('',#79217,#44796,#44797) ;
#35924=AXIS2_PLACEMENT_3D('',#79231,#44799,#44800) ;
#35925=AXIS2_PLACEMENT_3D('',#79256,#44801,#44802) ;
#35926=AXIS2_PLACEMENT_3D('',#79329,#44803,#44804) ;
#35927=AXIS2_PLACEMENT_3D('',#79402,#44805,#44806) ;
#35928=AXIS2_PLACEMENT_3D('',#79405,#44807,#44808) ;
#35929=AXIS2_PLACEMENT_3D('',#79409,#44810,#44811) ;
#35930=AXIS2_PLACEMENT_3D('',#79411,#44813,#44814) ;
#35931=AXIS2_PLACEMENT_3D('',#79414,#44815,#44816) ;
#35932=AXIS2_PLACEMENT_3D('',#79416,#44817,#44818) ;
#35933=AXIS2_PLACEMENT_3D('',#79418,#44819,#44820) ;
#35934=AXIS2_PLACEMENT_3D('',#79419,#44821,#44822) ;
#35935=AXIS2_PLACEMENT_3D('',#79420,#44823,#44824) ;
#35936=AXIS2_PLACEMENT_3D('',#79423,#44825,#44826) ;
#35937=AXIS2_PLACEMENT_3D('',#79426,#44829,#44830) ;
#35938=AXIS2_PLACEMENT_3D('',#79429,#44831,#44832) ;
#35939=AXIS2_PLACEMENT_3D('',#79431,#44833,#44834) ;
#35940=AXIS2_PLACEMENT_3D('',#79433,#44835,#44836) ;
#35941=AXIS2_PLACEMENT_3D('',#79434,#44837,#44838) ;
#35942=AXIS2_PLACEMENT_3D('',#79435,#44839,#44840) ;
#35943=AXIS2_PLACEMENT_3D('',#79438,#44841,#44842) ;
#35944=AXIS2_PLACEMENT_3D('',#79440,#44843,#44844) ;
#35945=AXIS2_PLACEMENT_3D('',#79442,#44845,#44846) ;
#35946=AXIS2_PLACEMENT_3D('',#79443,#44847,#44848) ;
#35947=AXIS2_PLACEMENT_3D('',#79444,#44849,#44850) ;
#35948=AXIS2_PLACEMENT_3D('',#79447,#44851,#44852) ;
#35949=AXIS2_PLACEMENT_3D('',#79450,#44855,#44856) ;
#35950=AXIS2_PLACEMENT_3D('',#79453,#44857,#44858) ;
#35951=AXIS2_PLACEMENT_3D('',#79454,#44859,#44860) ;
#35952=AXIS2_PLACEMENT_3D('',#79455,#44861,#44862) ;
#35953=AXIS2_PLACEMENT_3D('',#79456,#44863,#44864) ;
#35954=AXIS2_PLACEMENT_3D('',#79459,#44867,#44868) ;
#35955=AXIS2_PLACEMENT_3D('',#79461,#44869,#44870) ;
#35956=AXIS2_PLACEMENT_3D('',#79464,#44873,#44874) ;
#35957=AXIS2_PLACEMENT_3D('',#79467,#44875,#44876) ;
#35958=AXIS2_PLACEMENT_3D('',#79469,#44877,#44878) ;
#35959=AXIS2_PLACEMENT_3D('',#79471,#44879,#44880) ;
#35960=AXIS2_PLACEMENT_3D('',#79472,#44881,#44882) ;
#35961=AXIS2_PLACEMENT_3D('',#79473,#44883,#44884) ;
#35962=AXIS2_PLACEMENT_3D('',#79475,#44885,#44886) ;
#35963=AXIS2_PLACEMENT_3D('',#79478,#44889,#44890) ;
#35964=AXIS2_PLACEMENT_3D('',#79481,#44891,#44892) ;
#35965=AXIS2_PLACEMENT_3D('',#79484,#44895,#44896) ;
#35966=AXIS2_PLACEMENT_3D('',#79487,#44897,#44898) ;
#35967=AXIS2_PLACEMENT_3D('',#79488,#44899,#44900) ;
#35968=AXIS2_PLACEMENT_3D('',#79489,#44901,#44902) ;
#35969=AXIS2_PLACEMENT_3D('',#79490,#44903,#44904) ;
#35970=AXIS2_PLACEMENT_3D('',#79493,#44907,#44908) ;
#35971=AXIS2_PLACEMENT_3D('',#79496,#44911,#44912) ;
#35972=AXIS2_PLACEMENT_3D('',#79499,#44913,#44914) ;
#35973=AXIS2_PLACEMENT_3D('',#79502,#44917,#44918) ;
#35974=AXIS2_PLACEMENT_3D('',#79505,#44921,#44922) ;
#35975=AXIS2_PLACEMENT_3D('',#79506,#44923,#44924) ;
#35976=AXIS2_PLACEMENT_3D('',#79507,#44925,#44926) ;
#35977=AXIS2_PLACEMENT_3D('',#79508,#44927,#44928) ;
#35978=AXIS2_PLACEMENT_3D('',#79509,#44929,#44930) ;
#35979=AXIS2_PLACEMENT_3D('',#79511,#44931,#44932) ;
#35980=AXIS2_PLACEMENT_3D('',#79514,#44934,#44935) ;
#35981=AXIS2_PLACEMENT_3D('',#79516,#44937,#44938) ;
#35982=AXIS2_PLACEMENT_3D('',#79517,#44939,#44940) ;
#35983=AXIS2_PLACEMENT_3D('',#79518,#44941,#44942) ;
#35984=AXIS2_PLACEMENT_3D('',#79519,#44943,#44944) ;
#35985=AXIS2_PLACEMENT_3D('',#79520,#44945,#44946) ;
#35986=AXIS2_PLACEMENT_3D('',#79522,#44948,#44949) ;
#35987=AXIS2_PLACEMENT_3D('',#79526,#44951,#44952) ;
#35988=AXIS2_PLACEMENT_3D('',#79528,#44954,#44955) ;
#35989=AXIS2_PLACEMENT_3D('',#79542,#44958,#44959) ;
#35990=AXIS2_PLACEMENT_3D('',#79545,#44961,#44962) ;
#35991=AXIS2_PLACEMENT_3D('',#79546,#44963,#44964) ;
#35992=AXIS2_PLACEMENT_3D('',#79550,#44967,#44968) ;
#35993=AXIS2_PLACEMENT_3D('',#79551,#44969,#44970) ;
#35994=AXIS2_PLACEMENT_3D('',#79552,#44971,#44972) ;
#35995=AXIS2_PLACEMENT_3D('',#79554,#44974,#44975) ;
#35996=AXIS2_PLACEMENT_3D('',#79555,#44976,#44977) ;
#35997=AXIS2_PLACEMENT_3D('',#79558,#44979,#44980) ;
#35998=AXIS2_PLACEMENT_3D('',#79559,#44981,#44982) ;
#35999=AXIS2_PLACEMENT_3D('',#79563,#44984,#44985) ;
#36000=AXIS2_PLACEMENT_3D('',#79565,#44987,#44988) ;
#36001=AXIS2_PLACEMENT_3D('',#79567,#44989,#44990) ;
#36002=AXIS2_PLACEMENT_3D('',#79578,#44996,#44997) ;
#36003=AXIS2_PLACEMENT_3D('',#79579,#44998,#44999) ;
#36004=AXIS2_PLACEMENT_3D('',#79581,#45001,#45002) ;
#36005=AXIS2_PLACEMENT_3D('',#79600,#45007,#45008) ;
#36006=AXIS2_PLACEMENT_3D('',#79609,#45013,#45014) ;
#36007=AXIS2_PLACEMENT_3D('',#79616,#45017,#45018) ;
#36008=AXIS2_PLACEMENT_3D('',#79628,#45024,#45025) ;
#36009=AXIS2_PLACEMENT_3D('',#79630,#45027,#45028) ;
#36010=AXIS2_PLACEMENT_3D('',#79661,#45033,#45034) ;
#36011=AXIS2_PLACEMENT_3D('',#79662,#45035,#45036) ;
#36012=AXIS2_PLACEMENT_3D('',#79663,#45037,#45038) ;
#36013=AXIS2_PLACEMENT_3D('',#79664,#45039,#45040) ;
#36014=AXIS2_PLACEMENT_3D('',#79665,#45041,#45042) ;
#36015=AXIS2_PLACEMENT_3D('',#79666,#45043,#45044) ;
#36016=AXIS2_PLACEMENT_3D('',#79667,#45045,#45046) ;
#36017=AXIS2_PLACEMENT_3D('',#79695,#45048,#45049) ;
#36018=AXIS2_PLACEMENT_3D('',#79723,#45051,#45052) ;
#36019=AXIS2_PLACEMENT_3D('',#79732,#45057,#45058) ;
#36020=AXIS2_PLACEMENT_3D('',#79733,#45059,#45060) ;
#36021=AXIS2_PLACEMENT_3D('',#79734,#45061,#45062) ;
#36022=AXIS2_PLACEMENT_3D('',#79735,#45063,#45064) ;
#36023=AXIS2_PLACEMENT_3D('',#79742,#45067,#45068) ;
#36024=AXIS2_PLACEMENT_3D('',#79746,#45070,#45071) ;
#36025=AXIS2_PLACEMENT_3D('',#79748,#45073,#45074) ;
#36026=AXIS2_PLACEMENT_3D('',#79753,#45076,#45077) ;
#36027=AXIS2_PLACEMENT_3D('',#79757,#45079,#45080) ;
#36028=AXIS2_PLACEMENT_3D('',#79761,#45083,#45084) ;
#36029=AXIS2_PLACEMENT_3D('',#79763,#45085,#45086) ;
#36030=AXIS2_PLACEMENT_3D('',#79766,#45088,#45089) ;
#36031=AXIS2_PLACEMENT_3D('',#79767,#45090,#45091) ;
#36032=AXIS2_PLACEMENT_3D('',#79773,#45095,#45096) ;
#36033=AXIS2_PLACEMENT_3D('',#79775,#45097,#45098) ;
#36034=AXIS2_PLACEMENT_3D('',#79776,#45099,#45100) ;
#36035=AXIS2_PLACEMENT_3D('',#79777,#45101,#45102) ;
#36036=AXIS2_PLACEMENT_3D('',#79779,#45103,#45104) ;
#36037=AXIS2_PLACEMENT_3D('',#79780,#45105,#45106) ;
#36038=AXIS2_PLACEMENT_3D('',#79781,#45107,#45108) ;
#36039=AXIS2_PLACEMENT_3D('',#79783,#45109,#45110) ;
#36040=AXIS2_PLACEMENT_3D('',#79784,#45111,#45112) ;
#36041=AXIS2_PLACEMENT_3D('',#79785,#45113,#45114) ;
#36042=AXIS2_PLACEMENT_3D('',#79786,#45115,#45116) ;
#36043=AXIS2_PLACEMENT_3D('',#79787,#45117,#45118) ;
#36044=AXIS2_PLACEMENT_3D('',#79788,#45119,#45120) ;
#36045=AXIS2_PLACEMENT_3D('',#79790,#45121,#45122) ;
#36046=AXIS2_PLACEMENT_3D('',#79791,#45123,#45124) ;
#36047=AXIS2_PLACEMENT_3D('',#79792,#45125,#45126) ;
#36048=AXIS2_PLACEMENT_3D('',#79793,#45127,#45128) ;
#36049=AXIS2_PLACEMENT_3D('',#79794,#45129,#45130) ;
#36050=AXIS2_PLACEMENT_3D('',#79795,#45131,#45132) ;
#36051=AXIS2_PLACEMENT_3D('',#79796,#45133,#45134) ;
#36052=AXIS2_PLACEMENT_3D('',#79798,#45135,#45136) ;
#36053=AXIS2_PLACEMENT_3D('',#79800,#45138,#45139) ;
#36054=AXIS2_PLACEMENT_3D('',#79803,#45141,#45142) ;
#36055=AXIS2_PLACEMENT_3D('',#79804,#45143,#45144) ;
#36056=AXIS2_PLACEMENT_3D('',#79806,#45145,#45146) ;
#36057=AXIS2_PLACEMENT_3D('',#79808,#45148,#45149) ;
#36058=AXIS2_PLACEMENT_3D('',#79809,#45150,#45151) ;
#36059=AXIS2_PLACEMENT_3D('',#79810,#45152,#45153) ;
#36060=AXIS2_PLACEMENT_3D('',#79813,#45155,#45156) ;
#36061=AXIS2_PLACEMENT_3D('',#79814,#45157,#45158) ;
#36062=AXIS2_PLACEMENT_3D('',#79815,#45159,#45160) ;
#36063=AXIS2_PLACEMENT_3D('',#79816,#45161,#45162) ;
#36064=AXIS2_PLACEMENT_3D('',#79817,#45163,#45164) ;
#36065=AXIS2_PLACEMENT_3D('',#79818,#45165,#45166) ;
#36066=AXIS2_PLACEMENT_3D('',#79819,#45167,#45168) ;
#36067=AXIS2_PLACEMENT_3D('',#79820,#45169,#45170) ;
#36068=AXIS2_PLACEMENT_3D('',#79821,#45171,#45172) ;
#36069=AXIS2_PLACEMENT_3D('',#79822,#45173,#45174) ;
#36070=AXIS2_PLACEMENT_3D('',#79823,#45175,#45176) ;
#36071=AXIS2_PLACEMENT_3D('',#79824,#45177,#45178) ;
#36072=AXIS2_PLACEMENT_3D('',#79825,#45179,#45180) ;
#36073=AXIS2_PLACEMENT_3D('',#79827,#45181,#45182) ;
#36074=AXIS2_PLACEMENT_3D('',#79829,#45184,#45185) ;
#36075=AXIS2_PLACEMENT_3D('',#79830,#45186,#45187) ;
#36076=AXIS2_PLACEMENT_3D('',#79831,#45188,#45189) ;
#36077=AXIS2_PLACEMENT_3D('',#79834,#45191,#45192) ;
#36078=AXIS2_PLACEMENT_3D('',#79835,#45193,#45194) ;
#36079=AXIS2_PLACEMENT_3D('',#79836,#45195,#45196) ;
#36080=AXIS2_PLACEMENT_3D('',#79837,#45197,#45198) ;
#36081=AXIS2_PLACEMENT_3D('',#79838,#45199,#45200) ;
#36082=AXIS2_PLACEMENT_3D('',#79839,#45201,#45202) ;
#36083=AXIS2_PLACEMENT_3D('',#79840,#45203,#45204) ;
#36084=AXIS2_PLACEMENT_3D('',#79841,#45205,#45206) ;
#36085=AXIS2_PLACEMENT_3D('',#79842,#45207,#45208) ;
#36086=AXIS2_PLACEMENT_3D('',#79843,#45209,#45210) ;
#36087=AXIS2_PLACEMENT_3D('',#79844,#45211,#45212) ;
#36088=AXIS2_PLACEMENT_3D('',#79845,#45213,#45214) ;
#36089=AXIS2_PLACEMENT_3D('',#79846,#45215,#45216) ;
#36090=AXIS2_PLACEMENT_3D('',#79849,#45218,#45219) ;
#36091=AXIS2_PLACEMENT_3D('',#79850,#45220,#45221) ;
#36092=AXIS2_PLACEMENT_3D('',#79851,#45222,#45223) ;
#36093=AXIS2_PLACEMENT_3D('',#79852,#45224,#45225) ;
#36094=AXIS2_PLACEMENT_3D('',#79853,#45226,#45227) ;
#36095=AXIS2_PLACEMENT_3D('',#79854,#45228,#45229) ;
#36096=AXIS2_PLACEMENT_3D('',#79855,#45230,#45231) ;
#36097=AXIS2_PLACEMENT_3D('',#79856,#45232,#45233) ;
#36098=AXIS2_PLACEMENT_3D('',#79857,#45234,#45235) ;
#36099=AXIS2_PLACEMENT_3D('',#79858,#45236,#45237) ;
#36100=AXIS2_PLACEMENT_3D('',#79859,#45238,#45239) ;
#36101=AXIS2_PLACEMENT_3D('',#79860,#45240,#45241) ;
#36102=AXIS2_PLACEMENT_3D('',#79861,#45242,#45243) ;
#36103=AXIS2_PLACEMENT_3D('',#79862,#45244,#45245) ;
#36104=AXIS2_PLACEMENT_3D('',#79863,#45246,#45247) ;
#36105=AXIS2_PLACEMENT_3D('',#79864,#45248,#45249) ;
#36106=AXIS2_PLACEMENT_3D('',#79865,#45250,#45251) ;
#36107=AXIS2_PLACEMENT_3D('',#79867,#45252,#45253) ;
#36108=AXIS2_PLACEMENT_3D('',#79869,#45255,#45256) ;
#36109=AXIS2_PLACEMENT_3D('',#79870,#45257,#45258) ;
#36110=AXIS2_PLACEMENT_3D('',#79872,#45260,#45261) ;
#36111=AXIS2_PLACEMENT_3D('',#79873,#45262,#45263) ;
#36112=AXIS2_PLACEMENT_3D('',#79874,#45264,#45265) ;
#36113=AXIS2_PLACEMENT_3D('',#79875,#45266,#45267) ;
#36114=AXIS2_PLACEMENT_3D('',#79877,#45269,#45270) ;
#36115=AXIS2_PLACEMENT_3D('',#79878,#45271,#45272) ;
#36116=AXIS2_PLACEMENT_3D('',#79879,#45273,#45274) ;
#36117=AXIS2_PLACEMENT_3D('',#79880,#45275,#45276) ;
#36118=AXIS2_PLACEMENT_3D('',#79881,#45277,#45278) ;
#36119=AXIS2_PLACEMENT_3D('',#79882,#45279,#45280) ;
#36120=AXIS2_PLACEMENT_3D('',#79883,#45281,#45282) ;
#36121=AXIS2_PLACEMENT_3D('',#79884,#45283,#45284) ;
#36122=AXIS2_PLACEMENT_3D('',#79885,#45285,#45286) ;
#36123=AXIS2_PLACEMENT_3D('',#79887,#45287,#45288) ;
#36124=AXIS2_PLACEMENT_3D('',#79889,#45289,#45290) ;
#36125=AXIS2_PLACEMENT_3D('',#79890,#45291,#45292) ;
#36126=AXIS2_PLACEMENT_3D('',#79891,#45293,#45294) ;
#36127=AXIS2_PLACEMENT_3D('',#79893,#45295,#45296) ;
#36128=AXIS2_PLACEMENT_3D('',#79894,#45297,#45298) ;
#36129=AXIS2_PLACEMENT_3D('',#79897,#45299,#45300) ;
#36130=AXIS2_PLACEMENT_3D('',#79898,#45301,#45302) ;
#36131=AXIS2_PLACEMENT_3D('',#79900,#45304,#45305) ;
#36132=AXIS2_PLACEMENT_3D('',#79901,#45306,#45307) ;
#36133=AXIS2_PLACEMENT_3D('',#79902,#45308,#45309) ;
#44767=DIRECTION('axis',(0.,0.,1.)) ;
#44768=DIRECTION('refdir',(1.,0.,0.)) ;
#44769=DIRECTION('center_axis',(-3.59212155404594E-15,1.,1.73472347647041E-18)) ;
#44770=DIRECTION('ref_axis',(-2.70294271660742E-14,-1.7347234765675E-18,
1.)) ;
#44771=DIRECTION('',(-3.59212155404594E-15,1.,1.73472347647041E-18)) ;
#44772=DIRECTION('center_axis',(2.90739654573709E-15,-1.,2.17161023787725E-15)) ;
#44773=DIRECTION('ref_axis',(-2.70294271660742E-14,2.17161023787717E-15,
1.)) ;
#44774=DIRECTION('center_axis',(-3.59212155404594E-15,1.,1.73472347647041E-18)) ;
#44775=DIRECTION('ref_axis',(-2.70294271660742E-14,-1.7347234765675E-18,
1.)) ;
#44776=DIRECTION('',(-3.59212155404594E-15,1.,1.73472347647041E-18)) ;
#44777=DIRECTION('center_axis',(-3.59212155404594E-15,1.,1.73472347647041E-18)) ;
#44778=DIRECTION('ref_axis',(-2.70294271660742E-14,-1.7347234765675E-18,
1.)) ;
#44779=DIRECTION('',(-3.59212155404594E-15,1.,1.73472347647041E-18)) ;
#44780=DIRECTION('center_axis',(-3.59212155404594E-15,1.,1.73472347647041E-18)) ;
#44781=DIRECTION('ref_axis',(-2.70294271660742E-14,-1.7347234765675E-18,
1.)) ;
#44782=DIRECTION('',(-3.59212155404594E-15,1.,1.73472347647041E-18)) ;
#44783=DIRECTION('center_axis',(-2.9073965457371E-15,1.,-2.17161023787728E-15)) ;
#44784=DIRECTION('ref_axis',(-2.70294271660742E-14,2.1716102378772E-15,
1.)) ;
#44785=DIRECTION('center_axis',(-2.9073965457371E-15,1.,-2.17161023787728E-15)) ;
#44786=DIRECTION('ref_axis',(-1.48422940604576E-13,-2.17161023787771E-15,
-1.)) ;
#44787=DIRECTION('',(-2.9073965457371E-15,1.,-2.17161023787728E-15)) ;
#44788=DIRECTION('center_axis',(-2.90739654573709E-15,1.,-2.17161023787725E-15)) ;
#44789=DIRECTION('ref_axis',(-1.48422940604576E-13,-2.17161023787768E-15,
-1.)) ;
#44790=DIRECTION('center_axis',(-2.9073965457371E-15,1.,-2.17161023787728E-15)) ;
#44791=DIRECTION('ref_axis',(-1.48422940604576E-13,-2.17161023787771E-15,
-1.)) ;
#44792=DIRECTION('',(-2.9073965457371E-15,1.,-2.17161023787728E-15)) ;
#44793=DIRECTION('center_axis',(-2.9073965457371E-15,1.,-2.17161023787728E-15)) ;
#44794=DIRECTION('ref_axis',(-1.48422940604576E-13,-2.17161023787771E-15,
-1.)) ;
#44795=DIRECTION('',(-2.9073965457371E-15,1.,-2.17161023787728E-15)) ;
#44796=DIRECTION('center_axis',(-2.9073965457371E-15,1.,-2.17161023787728E-15)) ;
#44797=DIRECTION('ref_axis',(-1.48422940604576E-13,-2.17161023787771E-15,
-1.)) ;
#44798=DIRECTION('',(-2.9073965457371E-15,1.,-2.17161023787728E-15)) ;
#44799=DIRECTION('center_axis',(2.9073965457371E-15,-1.,2.17161023787728E-15)) ;
#44800=DIRECTION('ref_axis',(-1.48422940604576E-13,-2.17161023787771E-15,
-1.)) ;
#44801=DIRECTION('center_axis',(-2.9073965457371E-15,1.,-2.17161023787728E-15)) ;
#44802=DIRECTION('ref_axis',(-1.48422940604576E-13,-2.17161023787771E-15,
-1.)) ;
#44803=DIRECTION('center_axis',(-3.59212155404594E-15,1.,1.73472347647041E-18)) ;
#44804=DIRECTION('ref_axis',(-2.70294271660742E-14,-1.7347234765675E-18,
1.)) ;
#44805=DIRECTION('center_axis',(1.48422940604577E-13,2.17161023787771E-15,
1.)) ;
#44806=DIRECTION('ref_axis',(-0.707106781186548,-0.707106781186548,1.06486428110442E-13)) ;
#44807=DIRECTION('center_axis',(2.84217094304056E-13,0.,1.)) ;
#44808=DIRECTION('ref_axis',(-1.,0.,2.84217094304056E-13)) ;
#44809=DIRECTION('',(1.48422940604577E-13,2.17161023787771E-15,1.)) ;
#44810=DIRECTION('center_axis',(-2.84217094304016E-13,0.,-1.)) ;
#44811=DIRECTION('ref_axis',(0.,-1.,0.)) ;
#44812=DIRECTION('',(-1.48422940604577E-13,-2.17161023787771E-15,-1.)) ;
#44813=DIRECTION('center_axis',(-1.42108547152028E-13,0.,-1.)) ;
#44814=DIRECTION('ref_axis',(-1.,0.,1.81318720449162E-13)) ;
#44815=DIRECTION('center_axis',(5.59482469102649E-13,0.,-1.)) ;
#44816=DIRECTION('ref_axis',(0.,1.,0.)) ;
#44817=DIRECTION('center_axis',(1.,0.,-1.42108547152028E-13)) ;
#44818=DIRECTION('ref_axis',(1.42108547152028E-13,0.,1.)) ;
#44819=DIRECTION('center_axis',(1.48422940604576E-13,2.17161023787771E-15,
1.)) ;
#44820=DIRECTION('ref_axis',(-0.707106781186481,0.707106781186614,1.03415307459836E-13)) ;
#44821=DIRECTION('center_axis',(0.,-1.,0.)) ;
#44822=DIRECTION('ref_axis',(1.,0.,-2.84217094304056E-13)) ;
#44823=DIRECTION('center_axis',(-1.,-2.90739654573678E-15,1.48422940604576E-13)) ;
#44824=DIRECTION('ref_axis',(1.07006707598247E-13,-0.707106781186447,0.707106781186648)) ;
#44825=DIRECTION('center_axis',(-1.,0.,1.42108547152028E-13)) ;
#44826=DIRECTION('ref_axis',(0.,-1.,0.)) ;
#44827=DIRECTION('',(-1.,-2.90739654573678E-15,1.48422940604576E-13)) ;
#44828=DIRECTION('',(1.,2.90739654573678E-15,-1.48422940604576E-13)) ;
#44829=DIRECTION('center_axis',(1.42108547152028E-13,0.,1.)) ;
#44830=DIRECTION('ref_axis',(1.,0.,-1.81318720449162E-13)) ;
#44831=DIRECTION('center_axis',(0.,-5.59482469102493E-13,1.)) ;
#44832=DIRECTION('ref_axis',(-1.,0.,0.)) ;
#44833=DIRECTION('center_axis',(0.,-1.,0.)) ;
#44834=DIRECTION('ref_axis',(-1.42108547152069E-13,0.,-1.)) ;
#44835=DIRECTION('center_axis',(-1.48506207331423E-13,-2.17161023787768E-15,
-1.)) ;
#44836=DIRECTION('ref_axis',(-0.707106781186481,0.707106781186614,1.03474185927037E-13)) ;
#44837=DIRECTION('center_axis',(1.,0.,-1.42108547152028E-13)) ;
#44838=DIRECTION('ref_axis',(0.,-1.,0.)) ;
#44839=DIRECTION('center_axis',(-1.42108547152028E-13,0.,-1.)) ;
#44840=DIRECTION('ref_axis',(-1.,0.,1.81318720449162E-13)) ;
#44841=DIRECTION('center_axis',(0.,0.,-1.)) ;
#44842=DIRECTION('ref_axis',(1.,0.,0.)) ;
#44843=DIRECTION('center_axis',(0.,-1.,0.)) ;
#44844=DIRECTION('ref_axis',(1.42108547152028E-13,0.,1.)) ;
#44845=DIRECTION('center_axis',(1.48422940604576E-13,2.17161023787771E-15,
1.)) ;
#44846=DIRECTION('ref_axis',(0.707106781186481,0.707106781186614,-1.06486428110432E-13)) ;
#44847=DIRECTION('center_axis',(-1.,0.,1.42108547152028E-13)) ;
#44848=DIRECTION('ref_axis',(0.,-1.,0.)) ;
#44849=DIRECTION('center_axis',(2.90739654573712E-15,-1.,2.17161023787728E-15)) ;
#44850=DIRECTION('ref_axis',(-0.707106781186447,-5.20279487791395E-16,0.707106781186648)) ;
#44851=DIRECTION('center_axis',(0.,1.,0.)) ;
#44852=DIRECTION('ref_axis',(-1.,0.,2.84217094304097E-13)) ;
#44853=DIRECTION('',(-2.90739654573712E-15,1.,-2.17161023787728E-15)) ;
#44854=DIRECTION('',(2.90739654573712E-15,-1.,2.17161023787728E-15)) ;
#44855=DIRECTION('center_axis',(1.48422940604576E-13,2.17161023787771E-15,
1.)) ;
#44856=DIRECTION('ref_axis',(1.,0.,-1.79034390112784E-13)) ;
#44857=DIRECTION('center_axis',(0.,-1.,0.)) ;
#44858=DIRECTION('ref_axis',(1.,0.,-2.84217094304379E-13)) ;
#44859=DIRECTION('center_axis',(-1.48422940604576E-13,-2.17161023787771E-15,
-1.)) ;
#44860=DIRECTION('ref_axis',(-2.92171142922377E-14,-1.,2.17161023788205E-15)) ;
#44861=DIRECTION('center_axis',(1.48422940604576E-13,2.17161023787771E-15,
1.)) ;
#44862=DIRECTION('ref_axis',(-2.92171142922377E-14,-1.,2.17161023788205E-15)) ;
#44863=DIRECTION('center_axis',(-2.90739654573712E-15,1.,-2.17161023787728E-15)) ;
#44864=DIRECTION('ref_axis',(0.707106781186749,3.59140013838637E-15,0.707106781186347)) ;
#44865=DIRECTION('',(2.90739654573712E-15,-1.,2.17161023787728E-15)) ;
#44866=DIRECTION('',(-2.90739654573712E-15,1.,-2.17161023787728E-15)) ;
#44867=DIRECTION('center_axis',(-1.,-2.90739654573678E-15,1.48422940604576E-13)) ;
#44868=DIRECTION('ref_axis',(1.07006707598247E-13,-0.707106781186447,0.707106781186648)) ;
#44869=DIRECTION('center_axis',(1.,0.,-1.42108547151988E-13)) ;
#44870=DIRECTION('ref_axis',(1.42108547151988E-13,0.,1.)) ;
#44871=DIRECTION('',(1.,2.90739654573678E-15,-1.48422940604576E-13)) ;
#44872=DIRECTION('',(-1.,-2.90739654573678E-15,1.48422940604576E-13)) ;
#44873=DIRECTION('center_axis',(1.42108547152028E-13,0.,1.)) ;
#44874=DIRECTION('ref_axis',(1.,0.,-1.81318720449162E-13)) ;
#44875=DIRECTION('center_axis',(0.,0.,1.)) ;
#44876=DIRECTION('ref_axis',(0.,1.,0.)) ;
#44877=DIRECTION('center_axis',(-1.,0.,1.42108547152028E-13)) ;
#44878=DIRECTION('ref_axis',(-1.42108547152028E-13,0.,-1.)) ;
#44879=DIRECTION('center_axis',(-1.48506207331423E-13,-2.17161023787768E-15,
-1.)) ;
#44880=DIRECTION('ref_axis',(0.707106781186481,0.707106781186614,-1.06545306577632E-13)) ;
#44881=DIRECTION('center_axis',(0.,-1.,0.)) ;
#44882=DIRECTION('ref_axis',(-1.,0.,2.84217094304056E-13)) ;
#44883=DIRECTION('center_axis',(1.,2.90739654573678E-15,-1.48506207331423E-13)) ;
#44884=DIRECTION('ref_axis',(-1.02953906439241E-13,-0.707106781186648,-0.707106781186447)) ;
#44885=DIRECTION('center_axis',(1.,0.,-1.42108547152028E-13)) ;
#44886=DIRECTION('ref_axis',(0.,-1.,0.)) ;
#44887=DIRECTION('',(1.,2.90739654573678E-15,-1.48506207331423E-13)) ;
#44888=DIRECTION('',(-1.,-2.90739654573678E-15,1.48506207331423E-13)) ;
#44889=DIRECTION('center_axis',(2.90739654573712E-15,-1.,2.17161023787725E-15)) ;
#44890=DIRECTION('ref_axis',(0.707106781186447,5.20279487791416E-16,-0.707106781186648)) ;
#44891=DIRECTION('center_axis',(0.,1.,0.)) ;
#44892=DIRECTION('ref_axis',(1.,0.,-2.84217094303895E-13)) ;
#44893=DIRECTION('',(-2.90739654573712E-15,1.,-2.17161023787725E-15)) ;
#44894=DIRECTION('',(2.90739654573712E-15,-1.,2.17161023787725E-15)) ;
#44895=DIRECTION('center_axis',(-1.48506207331423E-13,-2.17161023787768E-15,
-1.)) ;
#44896=DIRECTION('ref_axis',(-1.,0.,1.79034390112784E-13)) ;
#44897=DIRECTION('center_axis',(0.,-1.,0.)) ;
#44898=DIRECTION('ref_axis',(-1.,0.,2.84217094303814E-13)) ;
#44899=DIRECTION('center_axis',(1.48506207331423E-13,2.17161023787768E-15,
1.)) ;
#44900=DIRECTION('ref_axis',(-2.67147415300443E-14,-1.,2.17161023788165E-15)) ;
#44901=DIRECTION('center_axis',(-1.48506207331423E-13,-2.17161023787768E-15,
-1.)) ;
#44902=DIRECTION('ref_axis',(-2.67147415300443E-14,-1.,2.17161023788165E-15)) ;
#44903=DIRECTION('center_axis',(-2.90739654573712E-15,1.,-2.17161023787725E-15)) ;
#44904=DIRECTION('ref_axis',(-0.707106781186648,-3.59140013838627E-15,-0.707106781186447)) ;
#44905=DIRECTION('',(2.90739654573712E-15,-1.,2.17161023787725E-15)) ;
#44906=DIRECTION('',(-2.90739654573712E-15,1.,-2.17161023787725E-15)) ;
#44907=DIRECTION('center_axis',(-1.48256407150882E-13,-2.17161023787771E-15,
-1.)) ;
#44908=DIRECTION('ref_axis',(0.707106781186548,0.707106781186548,-1.0636867117604E-13)) ;
#44909=DIRECTION('',(1.48256407150882E-13,2.17161023787771E-15,1.)) ;
#44910=DIRECTION('',(-1.48256407150882E-13,-2.17161023787771E-15,-1.)) ;
#44911=DIRECTION('center_axis',(1.,2.90739654573678E-15,-1.48506207331423E-13)) ;
#44912=DIRECTION('ref_axis',(-1.02953906439241E-13,-0.707106781186648,-0.707106781186447)) ;
#44913=DIRECTION('center_axis',(-1.,0.,1.42108547152028E-13)) ;
#44914=DIRECTION('ref_axis',(-1.42108547152028E-13,0.,-1.)) ;
#44915=DIRECTION('',(-1.,-2.90739654573678E-15,1.48506207331423E-13)) ;
#44916=DIRECTION('',(1.,2.90739654573678E-15,-1.48506207331423E-13)) ;
#44917=DIRECTION('center_axis',(1.48256407150882E-13,2.17161023787771E-15,
1.)) ;
#44918=DIRECTION('ref_axis',(-0.707106781186548,0.707106781186548,1.03297550525445E-13)) ;
#44919=DIRECTION('',(-1.48256407150882E-13,-2.17161023787771E-15,-1.)) ;
#44920=DIRECTION('',(1.48256407150882E-13,2.17161023787771E-15,1.)) ;
#44921=DIRECTION('center_axis',(0.408248290463711,0.408248290463711,-0.816496580927878)) ;
#44922=DIRECTION('ref_axis',(-0.577350269189815,-0.577350269189702,-0.57735026918936)) ;
#44923=DIRECTION('center_axis',(2.9073965457371E-15,-1.,2.17161023787725E-15)) ;
#44924=DIRECTION('ref_axis',(-0.707106781186619,-3.59140013838624E-15,-0.707106781186476)) ;
#44925=DIRECTION('center_axis',(0.408248290463901,-0.816496580927688,-0.408248290463901)) ;
#44926=DIRECTION('ref_axis',(-0.577350269189512,-0.577350269189626,0.57735026918974)) ;
#44927=DIRECTION('center_axis',(2.9073965457371E-15,-1.,2.17161023787728E-15)) ;
#44928=DIRECTION('ref_axis',(-0.707106781186334,-5.20279487790807E-16,0.707106781186761)) ;
#44929=DIRECTION('center_axis',(1.48422940604576E-13,2.17161023787771E-15,
1.)) ;
#44930=DIRECTION('ref_axis',(0.707106781186548,-0.707106781186548,-1.03415307459846E-13)) ;
#44931=DIRECTION('center_axis',(2.84217094304056E-13,0.,1.)) ;
#44932=DIRECTION('ref_axis',(0.,-1.,0.)) ;
#44933=DIRECTION('',(1.48422940604576E-13,2.17161023787771E-15,1.)) ;
#44934=DIRECTION('center_axis',(-2.84217094304056E-13,0.,-1.)) ;
#44935=DIRECTION('ref_axis',(1.,0.,-2.84217094304056E-13)) ;
#44936=DIRECTION('',(-1.48422940604576E-13,-2.17161023787771E-15,-1.)) ;
#44937=DIRECTION('center_axis',(-0.408248290463711,-0.816496580927764,0.408248290463939)) ;
#44938=DIRECTION('ref_axis',(0.57735026918955,-0.57735026918955,-0.577350269189777)) ;
#44939=DIRECTION('center_axis',(2.9073965457371E-15,-1.,2.17161023787725E-15)) ;
#44940=DIRECTION('ref_axis',(0.707106781186334,5.20279487790828E-16,-0.707106781186761)) ;
#44941=DIRECTION('center_axis',(0.408248290463901,-0.408248290463674,-0.816496580927802)) ;
#44942=DIRECTION('ref_axis',(0.57735026918974,-0.577350269189626,0.577350269189512)) ;
#44943=DIRECTION('center_axis',(2.9073965457371E-15,-1.,2.17161023787728E-15)) ;
#44944=DIRECTION('ref_axis',(0.707106781186619,3.59140013838626E-15,0.707106781186476)) ;
#44945=DIRECTION('center_axis',(-1.,-2.9073965457368E-15,1.48256407150882E-13)) ;
#44946=DIRECTION('ref_axis',(-2.90739654573712E-15,1.,-2.17161023787733E-15)) ;
#44947=DIRECTION('',(1.48256407150882E-13,2.17161023787776E-15,1.)) ;
#44948=DIRECTION('center_axis',(-2.9073965457371E-15,1.,-2.17161023787728E-15)) ;
#44949=DIRECTION('ref_axis',(-0.707106781186347,-5.20279487790871E-16,0.707106781186749)) ;
#44950=DIRECTION('',(-2.9073965457371E-15,1.,-2.17161023787728E-15)) ;
#44951=DIRECTION('center_axis',(-2.90739654573709E-15,1.,-2.17161023787725E-15)) ;
#44952=DIRECTION('ref_axis',(-1.,-2.90739654573647E-15,2.84217094304076E-13)) ;
#44953=DIRECTION('',(-2.9073965457371E-15,1.,-2.17161023787728E-15)) ;
#44954=DIRECTION('center_axis',(1.48422940604576E-13,2.17161023787771E-15,
1.)) ;
#44955=DIRECTION('ref_axis',(-1.,-2.90739654573678E-15,1.48422940604576E-13)) ;
#44956=DIRECTION('',(2.9073965457371E-15,-1.,2.17161023787728E-15)) ;
#44957=DIRECTION('',(1.,2.90739654573678E-15,-1.48422940604576E-13)) ;
#44958=DIRECTION('center_axis',(2.9073965457371E-15,-1.,2.17161023787728E-15)) ;
#44959=DIRECTION('ref_axis',(0.707106781186648,3.59140013838628E-15,0.707106781186447)) ;
#44960=DIRECTION('',(-2.9073965457371E-15,1.,-2.17161023787728E-15)) ;
#44961=DIRECTION('center_axis',(-2.90739654573709E-15,1.,-2.17161023787725E-15)) ;
#44962=DIRECTION('ref_axis',(1.,2.90739654573647E-15,-2.84217094304036E-13)) ;
#44963=DIRECTION('center_axis',(1.,2.90739654573678E-15,-1.48422940604576E-13)) ;
#44964=DIRECTION('ref_axis',(2.9073965457371E-15,-1.,2.17161023787728E-15)) ;
#44965=DIRECTION('',(2.9073965457371E-15,-1.,2.17161023787725E-15)) ;
#44966=DIRECTION('',(-1.48422940604576E-13,-2.17161023787768E-15,-1.)) ;
#44967=DIRECTION('center_axis',(2.9073965457371E-15,-1.,2.17161023787728E-15)) ;
#44968=DIRECTION('ref_axis',(1.48422940604576E-13,2.17161023787771E-15,
1.)) ;
#44969=DIRECTION('center_axis',(2.9073965457371E-15,-1.,2.17161023787728E-15)) ;
#44970=DIRECTION('ref_axis',(1.48422940604576E-13,2.17161023787771E-15,
1.)) ;
#44971=DIRECTION('center_axis',(1.,2.9073965457368E-15,-1.48256407150882E-13)) ;
#44972=DIRECTION('ref_axis',(2.90739654573712E-15,-1.,2.17161023787733E-15)) ;
#44973=DIRECTION('',(1.48256407150883E-13,2.17161023787776E-15,1.)) ;
#44974=DIRECTION('center_axis',(-1.48256407150882E-13,-2.17161023787776E-15,
-1.)) ;
#44975=DIRECTION('ref_axis',(1.,-2.20726215083294E-14,-1.48256407150882E-13)) ;
#44976=DIRECTION('center_axis',(-2.9073965457371E-15,1.,-2.17161023787725E-15)) ;
#44977=DIRECTION('ref_axis',(0.707106781186347,5.20279487790892E-16,-0.707106781186749)) ;
#44978=DIRECTION('',(-2.9073965457371E-15,1.,-2.17161023787725E-15)) ;
#44979=DIRECTION('center_axis',(-1.37109652768972E-44,-1.,2.17161023787773E-15)) ;
#44980=DIRECTION('ref_axis',(-1.42108547152028E-13,-2.17161023787773E-15,
-1.)) ;
#44981=DIRECTION('center_axis',(2.9073965457371E-15,-1.,2.17161023787725E-15)) ;
#44982=DIRECTION('ref_axis',(-0.707106781186648,-3.59140013838626E-15,-0.707106781186447)) ;
#44983=DIRECTION('',(-2.9073965457371E-15,1.,-2.17161023787725E-15)) ;
#44984=DIRECTION('center_axis',(-1.37109652768972E-44,-1.,2.17161023787773E-15)) ;
#44985=DIRECTION('ref_axis',(-1.,6.17208751770548E-28,2.84217094304056E-13)) ;
#44986=DIRECTION('',(2.9073965457371E-15,-1.,2.17161023787725E-15)) ;
#44987=DIRECTION('center_axis',(-1.48506207331423E-13,-2.17161023787768E-15,
-1.)) ;
#44988=DIRECTION('ref_axis',(1.,2.90739654573677E-15,-1.48506207331423E-13)) ;
#44989=DIRECTION('center_axis',(-1.48506207331423E-13,-2.17161023787768E-15,
-1.)) ;
#44990=DIRECTION('ref_axis',(0.707106781186497,0.707106781186598,-1.06545306577635E-13)) ;
#44991=DIRECTION('',(1.,2.90739654573677E-15,-1.48506207331423E-13)) ;
#44992=DIRECTION('',(2.90739654573709E-15,-1.,2.17161023787725E-15)) ;
#44993=DIRECTION('',(1.,2.90739654573677E-15,-1.48506207331423E-13)) ;
#44994=DIRECTION('',(-2.90739654573709E-15,1.,-2.17161023787725E-15)) ;
#44995=DIRECTION('',(1.,2.90739654573677E-15,-1.48506207331423E-13)) ;
#44996=DIRECTION('center_axis',(-1.48506207331423E-13,-2.17161023787768E-15,
-1.)) ;
#44997=DIRECTION('ref_axis',(-0.707106781186522,0.707106781186573,1.03474185927043E-13)) ;
#44998=DIRECTION('center_axis',(-1.,-2.90739654573678E-15,1.48422940604577E-13)) ;
#44999=DIRECTION('ref_axis',(2.9073965457371E-15,-1.,2.17161023787728E-15)) ;
#45000=DIRECTION('',(1.48422940604577E-13,2.17161023787768E-15,1.)) ;
#45001=DIRECTION('center_axis',(-1.48422940604576E-13,-2.17161023787771E-15,
-1.)) ;
#45002=DIRECTION('ref_axis',(1.,2.90739654573678E-15,-1.48422940604576E-13)) ;
#45003=DIRECTION('',(1.,2.90739654573678E-15,-1.48422940604576E-13)) ;
#45004=DIRECTION('',(2.9073965457371E-15,-1.,2.17161023787728E-15)) ;
#45005=DIRECTION('',(1.,2.90739654573678E-15,-1.48422940604576E-13)) ;
#45006=DIRECTION('',(-2.9073965457371E-15,1.,-2.17161023787728E-15)) ;
#45007=DIRECTION('center_axis',(2.9073965457371E-15,-1.,2.17161023787728E-15)) ;
#45008=DIRECTION('ref_axis',(1.48422940604576E-13,2.17161023787771E-15,
1.)) ;
#45009=DIRECTION('',(-1.,-2.90739654573678E-15,1.48422940604576E-13)) ;
#45010=DIRECTION('',(-1.48422940604576E-13,-2.17161023787771E-15,-1.)) ;
#45011=DIRECTION('',(1.,2.90739654573678E-15,-1.48506207331423E-13)) ;
#45012=DIRECTION('',(1.48422940604577E-13,2.17161023787771E-15,1.)) ;
#45013=DIRECTION('center_axis',(1.48506207331423E-13,2.17161023787768E-15,
1.)) ;
#45014=DIRECTION('ref_axis',(-1.,-2.90739654573677E-15,1.48506207331423E-13)) ;
#45015=DIRECTION('',(-1.,-2.90739654573678E-15,1.48506207331423E-13)) ;
#45016=DIRECTION('',(2.9073965457371E-15,-1.,2.17161023787725E-15)) ;
#45017=DIRECTION('center_axis',(1.48506207331423E-13,2.17161023787768E-15,
1.)) ;
#45018=DIRECTION('ref_axis',(-0.707106781186522,0.707106781186573,1.03474185927043E-13)) ;
#45019=DIRECTION('',(-1.,-2.90739654573677E-15,1.48506207331423E-13)) ;
#45020=DIRECTION('',(2.90739654573709E-15,-1.,2.17161023787725E-15)) ;
#45021=DIRECTION('',(1.,3.55570196157628E-15,-1.48506207331423E-13)) ;
#45022=DIRECTION('',(-2.90739654573709E-15,1.,-2.17161023787725E-15)) ;
#45023=DIRECTION('',(-1.,-2.90739654573677E-15,1.48506207331423E-13)) ;
#45024=DIRECTION('center_axis',(1.48506207331423E-13,2.17161023787768E-15,
1.)) ;
#45025=DIRECTION('ref_axis',(0.707106781186548,0.707106781186548,-1.06545306577642E-13)) ;
#45026=DIRECTION('',(-2.9073965457371E-15,1.,-2.17161023787725E-15)) ;
#45027=DIRECTION('center_axis',(-2.90739654573709E-15,1.,-2.17161023787725E-15)) ;
#45028=DIRECTION('ref_axis',(1.48506207331423E-13,2.17161023787768E-15,
1.)) ;
#45029=DIRECTION('',(-1.48506207331423E-13,-2.17161023787768E-15,-1.)) ;
#45030=DIRECTION('',(1.,2.90739654573677E-15,-1.48506207331423E-13)) ;
#45031=DIRECTION('',(1.48506207331423E-13,2.17161023787768E-15,1.)) ;
#45032=DIRECTION('',(1.,2.90739654573677E-15,-1.48506207331423E-13)) ;
#45033=DIRECTION('center_axis',(-1.,-2.90739654573677E-15,1.48506207331423E-13)) ;
#45034=DIRECTION('ref_axis',(1.02953906439256E-13,0.707106781186549,0.707106781186546)) ;
#45035=DIRECTION('center_axis',(-1.,-2.90739654573677E-15,1.48506207331423E-13)) ;
#45036=DIRECTION('ref_axis',(1.02953906439256E-13,0.707106781186543,0.707106781186552)) ;
#45037=DIRECTION('center_axis',(1.,2.90739654573677E-15,-1.48506207331423E-13)) ;
#45038=DIRECTION('ref_axis',(1.02953906439253E-13,0.707106781186567,0.707106781186528)) ;
#45039=DIRECTION('center_axis',(-1.,-2.90739654573677E-15,1.48506207331423E-13)) ;
#45040=DIRECTION('ref_axis',(-1.07065586065433E-13,0.707106781186549,-0.707106781186546)) ;
#45041=DIRECTION('center_axis',(-1.,-2.90739654573677E-15,1.48506207331423E-13)) ;
#45042=DIRECTION('ref_axis',(-1.07065586065431E-13,0.707106781186565,-0.70710678118653)) ;
#45043=DIRECTION('center_axis',(1.,2.90739654573677E-15,-1.48506207331423E-13)) ;
#45044=DIRECTION('ref_axis',(-1.07065586065434E-13,0.70710678118654,-0.707106781186555)) ;
#45045=DIRECTION('center_axis',(1.,2.90739654573678E-15,-1.48422940604576E-13)) ;
#45046=DIRECTION('ref_axis',(1.02895027972065E-13,0.707106781186482,0.707106781186613)) ;
#45047=DIRECTION('',(-1.,-2.90739654573678E-15,1.48422940604576E-13)) ;
#45048=DIRECTION('center_axis',(1.,2.90739654573678E-15,-1.48422940604576E-13)) ;
#45049=DIRECTION('ref_axis',(-1.07006707598192E-13,0.707106781186829,-0.707106781186266)) ;
#45050=DIRECTION('',(-1.,-2.90739654573678E-15,1.48422940604576E-13)) ;
#45051=DIRECTION('center_axis',(1.,2.90739654573678E-15,-1.48422940604576E-13)) ;
#45052=DIRECTION('ref_axis',(2.9073965457371E-15,-1.,2.17161023787728E-15)) ;
#45053=DIRECTION('',(1.48422940604576E-13,2.17161023787771E-15,1.)) ;
#45054=DIRECTION('',(2.9073965457371E-15,-1.,2.17161023787728E-15)) ;
#45055=DIRECTION('',(-1.48422940604576E-13,-2.17161023787768E-15,-1.)) ;
#45056=DIRECTION('',(-2.9073965457371E-15,1.,-2.17161023787725E-15)) ;
#45057=DIRECTION('center_axis',(-2.9073965457371E-15,1.,-2.17161023787728E-15)) ;
#45058=DIRECTION('ref_axis',(0.707106781186347,5.20279487790871E-16,-0.707106781186749)) ;
#45059=DIRECTION('center_axis',(2.9073965457371E-15,-1.,2.17161023787728E-15)) ;
#45060=DIRECTION('ref_axis',(0.707106781186334,5.20279487790807E-16,-0.707106781186761)) ;
#45061=DIRECTION('center_axis',(-2.90739654573709E-15,1.,-2.17161023787725E-15)) ;
#45062=DIRECTION('ref_axis',(1.,2.90739654573647E-15,-2.84217094304056E-13)) ;
#45063=DIRECTION('center_axis',(1.,2.90739654573677E-15,-1.48506207331423E-13)) ;
#45064=DIRECTION('ref_axis',(2.90739654573709E-15,-1.,2.17161023787725E-15)) ;
#45065=DIRECTION('',(1.48506207331423E-13,2.17161023787768E-15,1.)) ;
#45066=DIRECTION('',(2.90739654573709E-15,-1.,2.17161023787725E-15)) ;
#45067=DIRECTION('center_axis',(-1.,-2.90739654573677E-15,1.48506207331423E-13)) ;
#45068=DIRECTION('ref_axis',(-1.07065586065434E-13,0.70710678118654,-0.707106781186555)) ;
#45069=DIRECTION('',(-1.48506207331423E-13,-2.17161023787768E-15,-1.)) ;
#45070=DIRECTION('center_axis',(-1.,-2.90739654573677E-15,1.48506207331423E-13)) ;
#45071=DIRECTION('ref_axis',(1.02953906439253E-13,0.707106781186567,0.707106781186528)) ;
#45072=DIRECTION('',(-2.90739654573709E-15,1.,-2.17161023787725E-15)) ;
#45073=DIRECTION('center_axis',(-1.,-2.90739654573677E-15,1.48506207331423E-13)) ;
#45074=DIRECTION('ref_axis',(2.90739654573709E-15,-1.,2.17161023787725E-15)) ;
#45075=DIRECTION('',(2.90739654573709E-15,-1.,2.17161023787725E-15)) ;
#45076=DIRECTION('center_axis',(1.,2.90739654573677E-15,-1.48506207331423E-13)) ;
#45077=DIRECTION('ref_axis',(1.02953906439256E-13,0.707106781186544,0.707106781186551)) ;
#45078=DIRECTION('',(1.48506207331423E-13,2.17161023787768E-15,1.)) ;
#45079=DIRECTION('center_axis',(1.,2.90739654573677E-15,-1.48506207331423E-13)) ;
#45080=DIRECTION('ref_axis',(-1.07065586065431E-13,0.707106781186565,-0.70710678118653)) ;
#45081=DIRECTION('',(-2.90739654573709E-15,1.,-2.17161023787725E-15)) ;
#45082=DIRECTION('',(-1.48506207331423E-13,-2.17161023787768E-15,-1.)) ;
#45083=DIRECTION('center_axis',(2.9073965457371E-15,-1.,2.17161023787728E-15)) ;
#45084=DIRECTION('ref_axis',(-0.707106781186749,-3.59140013838635E-15,-0.707106781186347)) ;
#45085=DIRECTION('center_axis',(2.9073965457371E-15,-1.,2.17161023787728E-15)) ;
#45086=DIRECTION('ref_axis',(-0.70710678118669,-3.59140013838631E-15,-0.707106781186405)) ;
#45087=DIRECTION('',(-2.9073965457371E-15,1.,-2.17161023787728E-15)) ;
#45088=DIRECTION('center_axis',(-2.90739654573709E-15,1.,-2.17161023787725E-15)) ;
#45089=DIRECTION('ref_axis',(-1.,-2.90739654573647E-15,2.84217094304056E-13)) ;
#45090=DIRECTION('center_axis',(-1.,-2.90739654573678E-15,1.48422940604577E-13)) ;
#45091=DIRECTION('ref_axis',(2.9073965457371E-15,-1.,2.17161023787728E-15)) ;
#45092=DIRECTION('',(-1.48422940604577E-13,-2.17161023787771E-15,-1.)) ;
#45093=DIRECTION('',(2.9073965457371E-15,-1.,2.17161023787725E-15)) ;
#45094=DIRECTION('',(1.48422940604577E-13,2.17161023787768E-15,1.)) ;
#45095=DIRECTION('center_axis',(2.90739654573709E-15,-1.,2.17161023787725E-15)) ;
#45096=DIRECTION('ref_axis',(0.414201389893284,0.,0.910185260598342)) ;
#45097=DIRECTION('center_axis',(2.84217094304016E-13,2.17161023787773E-15,
1.)) ;
#45098=DIRECTION('ref_axis',(0.,1.,-2.17161023787773E-15)) ;
#45099=DIRECTION('center_axis',(2.90739654573709E-15,-1.,2.17161023787725E-15)) ;
#45100=DIRECTION('ref_axis',(1.,2.90739654573647E-15,-2.84217094304036E-13)) ;
#45101=DIRECTION('center_axis',(2.90739654573709E-15,-1.,2.17161023787725E-15)) ;
#45102=DIRECTION('ref_axis',(-0.41420138989285,0.,0.910185260598539)) ;
#45103=DIRECTION('center_axis',(2.90739654573709E-15,-1.,2.17161023787725E-15)) ;
#45104=DIRECTION('ref_axis',(-1.,-2.90739654573647E-15,2.84217094304076E-13)) ;
#45105=DIRECTION('center_axis',(2.84217094304056E-13,2.17161023787773E-15,
1.)) ;
#45106=DIRECTION('ref_axis',(1.,-6.17208751770549E-28,-2.84217094304056E-13)) ;
#45107=DIRECTION('center_axis',(2.90739654573709E-15,-1.,2.17161023787725E-15)) ;
#45108=DIRECTION('ref_axis',(0.,0.,-1.)) ;
#45109=DIRECTION('center_axis',(2.90739654573709E-15,-1.,2.17161023787725E-15)) ;
#45110=DIRECTION('ref_axis',(1.,2.90739654573647E-15,-2.84217094304056E-13)) ;
#45111=DIRECTION('center_axis',(-2.84217094304016E-13,-2.17161023787773E-15,
-1.)) ;
#45112=DIRECTION('ref_axis',(-1.,6.17208751770461E-28,2.84217094304016E-13)) ;
#45113=DIRECTION('center_axis',(0.408248290463711,0.408248290463711,-0.816496580927878)) ;
#45114=DIRECTION('ref_axis',(-0.577350269189815,-0.577350269189702,-0.57735026918936)) ;
#45115=DIRECTION('center_axis',(2.84217094304056E-13,2.17161023787773E-15,
1.)) ;
#45116=DIRECTION('ref_axis',(-1.,6.17208751770549E-28,2.84217094304056E-13)) ;
#45117=DIRECTION('center_axis',(1.,-3.08604375885274E-28,-1.42108547152028E-13)) ;
#45118=DIRECTION('ref_axis',(1.04928462787225E-43,-1.,2.17161023787773E-15)) ;
#45119=DIRECTION('center_axis',(2.90739654573709E-15,-1.,2.17161023787725E-15)) ;
#45120=DIRECTION('ref_axis',(0.,0.,-1.)) ;
#45121=DIRECTION('center_axis',(-2.84217094304097E-13,-2.17161023787773E-15,
-1.)) ;
#45122=DIRECTION('ref_axis',(0.,1.,-2.17161023787773E-15)) ;
#45123=DIRECTION('center_axis',(2.90739654573709E-15,-1.,2.17161023787725E-15)) ;
#45124=DIRECTION('ref_axis',(-1.,-2.90739654573647E-15,2.84217094304056E-13)) ;
#45125=DIRECTION('center_axis',(-0.408248290463711,-0.816496580927764,0.408248290463939)) ;
#45126=DIRECTION('ref_axis',(0.577350269189474,-0.577350269189474,-0.577350269189929)) ;
#45127=DIRECTION('center_axis',(-1.,3.08604375885274E-28,1.42108547152028E-13)) ;
#45128=DIRECTION('ref_axis',(-1.42108547152028E-13,-2.17161023787773E-15,
-1.)) ;
#45129=DIRECTION('center_axis',(2.84217094304056E-13,2.17161023787773E-15,
1.)) ;
#45130=DIRECTION('ref_axis',(0.,-1.,2.17161023787773E-15)) ;
#45131=DIRECTION('center_axis',(1.,2.90739654573678E-15,-1.48422940604576E-13)) ;
#45132=DIRECTION('ref_axis',(-1.02895027972062E-13,-0.707106781186499,-0.707106781186596)) ;
#45133=DIRECTION('center_axis',(-1.48422940604576E-13,-2.17161023787768E-15,
-1.)) ;
#45134=DIRECTION('ref_axis',(-0.707106781186497,0.707106781186598,1.03415307459839E-13)) ;
#45135=DIRECTION('center_axis',(2.84217094304056E-13,-2.82045484066158E-13,
1.)) ;
#45136=DIRECTION('ref_axis',(-1.,6.17208751770553E-28,2.84217094304056E-13)) ;
#45137=DIRECTION('',(1.48422940604576E-13,2.17161023787768E-15,1.)) ;
#45138=DIRECTION('center_axis',(1.48422940604577E-13,2.17161023787768E-15,
1.)) ;
#45139=DIRECTION('ref_axis',(0.707106781186548,0.707106781186548,-1.06486428110442E-13)) ;
#45140=DIRECTION('',(-1.48422940604577E-13,-2.17161023787768E-15,-1.)) ;
#45141=DIRECTION('center_axis',(-6.31373210429172E-30,2.17161023787773E-15,
1.)) ;
#45142=DIRECTION('ref_axis',(1.37109652768972E-44,1.,-2.17161023787773E-15)) ;
#45143=DIRECTION('center_axis',(1.,2.90739654573677E-15,-1.48506207331423E-13)) ;
#45144=DIRECTION('ref_axis',(-1.02953906439233E-13,-0.7071067811867,-0.707106781186395)) ;
#45145=DIRECTION('center_axis',(1.,-3.08604375885274E-28,-1.42108547152028E-13)) ;
#45146=DIRECTION('ref_axis',(-1.42108547152028E-13,-2.17161023787773E-15,
-1.)) ;
#45147=DIRECTION('',(-1.,-2.90739654573677E-15,1.48506207331423E-13)) ;
#45148=DIRECTION('center_axis',(1.,-3.08604375885274E-28,-1.42108547152028E-13)) ;
#45149=DIRECTION('ref_axis',(1.04928462787225E-43,-1.,2.17161023787773E-15)) ;
#45150=DIRECTION('center_axis',(1.,2.90739654573677E-15,-1.48506207331423E-13)) ;
#45151=DIRECTION('ref_axis',(-1.02953906439233E-13,-0.7071067811867,-0.707106781186395)) ;
#45152=DIRECTION('center_axis',(-1.,3.08604375885274E-28,1.42108547152028E-13)) ;
#45153=DIRECTION('ref_axis',(-1.42108547152028E-13,-2.17161023787773E-15,
-1.)) ;
#45154=DIRECTION('',(-1.,-2.90739654573677E-15,1.48506207331423E-13)) ;
#45155=DIRECTION('center_axis',(-1.,6.17208751770549E-28,2.84217094304056E-13)) ;
#45156=DIRECTION('ref_axis',(-7.76657193310222E-43,-1.,2.17161023787773E-15)) ;
#45157=DIRECTION('center_axis',(2.90739654573709E-15,-1.,2.17161023787725E-15)) ;
#45158=DIRECTION('ref_axis',(0.707106781186749,3.59140013838632E-15,0.707106781186347)) ;
#45159=DIRECTION('center_axis',(-1.37109652768972E-44,-1.,2.17161023787773E-15)) ;
#45160=DIRECTION('ref_axis',(1.42108547152028E-13,2.17161023787773E-15,
1.)) ;
#45161=DIRECTION('center_axis',(1.37109652768972E-44,1.,-2.17161023787773E-15)) ;
#45162=DIRECTION('ref_axis',(2.84217094304056E-13,2.17161023787773E-15,
1.)) ;
#45163=DIRECTION('center_axis',(-1.,-2.90739654573677E-15,1.48506207331423E-13)) ;
#45164=DIRECTION('ref_axis',(1.62758536466166E-13,0.,1.)) ;
#45165=DIRECTION('center_axis',(-2.84217094304016E-13,-2.17161023787773E-15,
-1.)) ;
#45166=DIRECTION('ref_axis',(0.,1.,-2.17161023787773E-15)) ;
#45167=DIRECTION('center_axis',(1.48506207331423E-13,2.17161023787768E-15,
1.)) ;
#45168=DIRECTION('ref_axis',(0.707106781186648,0.707106781186447,-1.06545306577657E-13)) ;
#45169=DIRECTION('center_axis',(-2.84217094304056E-13,-2.17161023787773E-15,
-1.)) ;
#45170=DIRECTION('ref_axis',(0.,1.,-2.17161023787773E-15)) ;
#45171=DIRECTION('center_axis',(-1.,-2.90739654573677E-15,1.48506207331423E-13)) ;
#45172=DIRECTION('ref_axis',(1.62758536466166E-13,0.,1.)) ;
#45173=DIRECTION('center_axis',(-1.37109652768972E-44,-1.,2.17161023787773E-15)) ;
#45174=DIRECTION('ref_axis',(-1.42108547152069E-13,-2.17161023787773E-15,
-1.)) ;
#45175=DIRECTION('center_axis',(-2.90739654573709E-15,1.,-2.17161023787725E-15)) ;
#45176=DIRECTION('ref_axis',(0.707106781186347,5.20279487790885E-16,-0.707106781186749)) ;
#45177=DIRECTION('center_axis',(-4.03896783473261E-26,-1.,-1.3993693691415E-13)) ;
#45178=DIRECTION('ref_axis',(1.,-6.17208751770659E-28,-2.84217094304097E-13)) ;
#45179=DIRECTION('center_axis',(1.48506207331423E-13,2.17161023787768E-15,
1.)) ;
#45180=DIRECTION('ref_axis',(0.707106781186548,-0.707106781186548,-1.03474185927047E-13)) ;
#45181=DIRECTION('center_axis',(2.84217094304056E-13,2.17161023787773E-15,
1.)) ;
#45182=DIRECTION('ref_axis',(1.,-6.17208751770549E-28,-2.84217094304056E-13)) ;
#45183=DIRECTION('',(-1.48506207331423E-13,-2.17161023787768E-15,-1.)) ;
#45184=DIRECTION('center_axis',(-2.84217094304056E-13,-2.17161023787773E-15,
-1.)) ;
#45185=DIRECTION('ref_axis',(0.,-1.,2.17161023787773E-15)) ;
#45186=DIRECTION('center_axis',(-1.48506207331423E-13,-2.17161023787768E-15,
-1.)) ;
#45187=DIRECTION('ref_axis',(-0.707106781186497,-0.707106781186598,1.06545306577635E-13)) ;
#45188=DIRECTION('center_axis',(-2.84217094304056E-13,-2.17161023787773E-15,
-1.)) ;
#45189=DIRECTION('ref_axis',(-1.,6.17208751770549E-28,2.84217094304056E-13)) ;
#45190=DIRECTION('',(1.48506207331423E-13,2.17161023787768E-15,1.)) ;
#45191=DIRECTION('center_axis',(2.84217094304056E-13,2.17161023787773E-15,
1.)) ;
#45192=DIRECTION('ref_axis',(0.,-1.,2.17161023787773E-15)) ;
#45193=DIRECTION('center_axis',(2.90739654573709E-15,-1.,2.17161023787725E-15)) ;
#45194=DIRECTION('ref_axis',(-0.707106781186648,-3.59140013838625E-15,-0.707106781186447)) ;
#45195=DIRECTION('center_axis',(7.10542735760242E-14,-1.,2.17161023786763E-15)) ;
#45196=DIRECTION('ref_axis',(-1.42108547152028E-13,-2.17161023787773E-15,
-1.)) ;
#45197=DIRECTION('center_axis',(1.37109652768972E-44,1.,-2.17161023787773E-15)) ;
#45198=DIRECTION('ref_axis',(-2.84217094304056E-13,-2.17161023787773E-15,
-1.)) ;
#45199=DIRECTION('center_axis',(1.,2.90739654573677E-15,-1.48506207331423E-13)) ;
#45200=DIRECTION('ref_axis',(-1.42413719407895E-13,0.,-1.)) ;
#45201=DIRECTION('center_axis',(2.84217094304056E-13,2.17161023787773E-15,
1.)) ;
#45202=DIRECTION('ref_axis',(0.,1.,-2.17161023787773E-15)) ;
#45203=DIRECTION('center_axis',(1.48506207331423E-13,2.17161023787768E-15,
1.)) ;
#45204=DIRECTION('ref_axis',(-0.707106781186548,0.707106781186548,1.03474185927047E-13)) ;
#45205=DIRECTION('center_axis',(2.84217094304056E-13,-2.82045484066138E-13,
1.)) ;
#45206=DIRECTION('ref_axis',(0.,1.,2.82045484066138E-13)) ;
#45207=DIRECTION('center_axis',(1.,2.90739654573677E-15,-1.48506207331423E-13)) ;
#45208=DIRECTION('ref_axis',(-1.42413719407895E-13,0.,-1.)) ;
#45209=DIRECTION('center_axis',(-1.37109652768972E-44,-1.,2.17161023787773E-15)) ;
#45210=DIRECTION('ref_axis',(1.42108547152069E-13,2.17161023787773E-15,
1.)) ;
#45211=DIRECTION('center_axis',(-2.90739654573709E-15,1.,-2.17161023787725E-15)) ;
#45212=DIRECTION('ref_axis',(-0.707106781186447,-5.20279487791395E-16,0.707106781186648)) ;
#45213=DIRECTION('center_axis',(-2.01948391736573E-26,-1.,-6.88826633381363E-14)) ;
#45214=DIRECTION('ref_axis',(-1.,6.1720875177043E-28,2.84217094304016E-13)) ;
#45215=DIRECTION('center_axis',(-1.48422940604576E-13,-2.17161023787768E-15,
-1.)) ;
#45216=DIRECTION('ref_axis',(-0.707106781186497,0.707106781186598,1.03415307459839E-13)) ;
#45217=DIRECTION('',(1.48422940604576E-13,2.17161023787768E-15,1.)) ;
#45218=DIRECTION('center_axis',(6.31373210429172E-30,-2.17161023787773E-15,
-1.)) ;
#45219=DIRECTION('ref_axis',(1.37109652768972E-44,1.,-2.17161023787773E-15)) ;
#45220=DIRECTION('center_axis',(2.9073965457371E-15,-1.,2.17161023787725E-15)) ;
#45221=DIRECTION('ref_axis',(0.707106781186749,3.59140013838633E-15,0.707106781186347)) ;
#45222=DIRECTION('center_axis',(-7.10542735760141E-14,-1.,2.17161023788783E-15)) ;
#45223=DIRECTION('ref_axis',(1.42108547152028E-13,2.17161023787773E-15,
1.)) ;
#45224=DIRECTION('center_axis',(-1.37109652768972E-44,-1.,2.17161023787773E-15)) ;
#45225=DIRECTION('ref_axis',(1.,-6.17208751770548E-28,-2.84217094304056E-13)) ;
#45226=DIRECTION('center_axis',(1.48422940604576E-13,2.17161023787771E-15,
1.)) ;
#45227=DIRECTION('ref_axis',(0.707106781186497,-0.707106781186598,-1.03415307459839E-13)) ;
#45228=DIRECTION('center_axis',(2.84217094304056E-13,2.17161023787773E-15,
1.)) ;
#45229=DIRECTION('ref_axis',(1.,-6.17208751770549E-28,-2.84217094304056E-13)) ;
#45230=DIRECTION('center_axis',(-1.48422940604577E-13,-2.17161023787771E-15,
-1.)) ;
#45231=DIRECTION('ref_axis',(-0.707106781186497,-0.707106781186598,1.06486428110435E-13)) ;
#45232=DIRECTION('center_axis',(2.84217094304056E-13,2.17161023787773E-15,
1.)) ;
#45233=DIRECTION('ref_axis',(0.,-1.,2.17161023787773E-15)) ;
#45234=DIRECTION('center_axis',(-2.9073965457371E-15,1.,-2.17161023787725E-15)) ;
#45235=DIRECTION('ref_axis',(-0.707106781186447,-5.20279487791402E-16,0.707106781186648)) ;
#45236=DIRECTION('center_axis',(-1.37109652768972E-44,-1.,2.17161023787773E-15)) ;
#45237=DIRECTION('ref_axis',(1.42108547152028E-13,2.17161023787773E-15,
1.)) ;
#45238=DIRECTION('center_axis',(-1.37109652768972E-44,-1.,2.17161023787773E-15)) ;
#45239=DIRECTION('ref_axis',(-1.,6.17208751770548E-28,2.84217094304056E-13)) ;
#45240=DIRECTION('center_axis',(-1.,-2.90739654573678E-15,1.48506207331423E-13)) ;
#45241=DIRECTION('ref_axis',(1.07065586065441E-13,-0.707106781186496,0.707106781186599)) ;
#45242=DIRECTION('center_axis',(1.,-3.08604375885274E-28,-1.42108547152028E-13)) ;
#45243=DIRECTION('ref_axis',(1.04928462787225E-43,-1.,2.17161023787773E-15)) ;
#45244=DIRECTION('center_axis',(-1.,3.08604375885274E-28,1.42108547152028E-13)) ;
#45245=DIRECTION('ref_axis',(1.42108547152028E-13,2.17161023787773E-15,
1.)) ;
#45246=DIRECTION('center_axis',(0.408248290463711,-0.816496580927764,-0.408248290463939)) ;
#45247=DIRECTION('ref_axis',(-0.57735026918955,-0.57735026918955,0.577350269189777)) ;
#45248=DIRECTION('center_axis',(-0.816496580927688,-0.408248290463958,0.408248290463844)) ;
#45249=DIRECTION('ref_axis',(0.577350269189702,-0.577350269189702,0.577350269189474)) ;
#45250=DIRECTION('center_axis',(1.48422940604577E-13,2.17161023787768E-15,
1.)) ;
#45251=DIRECTION('ref_axis',(0.707106781186548,0.707106781186548,-1.06486428110442E-13)) ;
#45252=DIRECTION('center_axis',(-2.84217094304056E-13,-2.86388704541914E-13,
-1.)) ;
#45253=DIRECTION('ref_axis',(1.,-6.17208751770544E-28,-2.84217094304056E-13)) ;
#45254=DIRECTION('',(-1.48422940604577E-13,-2.17161023787768E-15,-1.)) ;
#45255=DIRECTION('center_axis',(-1.,-2.90739654573677E-15,1.48506207331423E-13)) ;
#45256=DIRECTION('ref_axis',(1.07065586065419E-13,-0.707106781186646,0.707106781186449)) ;
#45257=DIRECTION('center_axis',(-1.,2.84217094304057E-13,1.42108547152027E-13)) ;
#45258=DIRECTION('ref_axis',(1.42108547152028E-13,2.17161023787773E-15,
1.)) ;
#45259=DIRECTION('',(1.,2.90739654573677E-15,-1.48506207331423E-13)) ;
#45260=DIRECTION('center_axis',(-1.,3.08604375885274E-28,1.42108547152028E-13)) ;
#45261=DIRECTION('ref_axis',(1.04928462787225E-43,-1.,2.17161023787773E-15)) ;
#45262=DIRECTION('center_axis',(1.42108547152028E-13,2.17161023787773E-15,
1.)) ;
#45263=DIRECTION('ref_axis',(1.,0.,-1.51582450295488E-13)) ;
#45264=DIRECTION('center_axis',(-1.,-2.90739654573677E-15,1.48506207331423E-13)) ;
#45265=DIRECTION('ref_axis',(1.07065586065419E-13,-0.707106781186646,0.707106781186449)) ;
#45266=DIRECTION('center_axis',(1.,-3.08604375885274E-28,-1.42108547152028E-13)) ;
#45267=DIRECTION('ref_axis',(1.42108547152028E-13,2.17161023787773E-15,
1.)) ;
#45268=DIRECTION('',(1.,2.90739654573677E-15,-1.48506207331423E-13)) ;
#45269=DIRECTION('center_axis',(1.,0.,6.31373210429172E-30)) ;
#45270=DIRECTION('ref_axis',(-1.37109652768972E-44,-1.,2.17161023787773E-15)) ;
#45271=DIRECTION('center_axis',(-1.42108547152028E-13,-2.17161023787773E-15,
-1.)) ;
#45272=DIRECTION('ref_axis',(-1.,0.,1.51582450295488E-13)) ;
#45273=DIRECTION('center_axis',(-0.408248290463958,-0.408248290463844,-0.816496580927688)) ;
#45274=DIRECTION('ref_axis',(-0.577350269189815,-0.577350269189474,0.577350269189588)) ;
#45275=DIRECTION('center_axis',(-0.816496580927726,-0.408248290463977,0.408248290463749)) ;
#45276=DIRECTION('ref_axis',(0.577350269189588,-0.577350269189702,0.577350269189588)) ;
#45277=DIRECTION('center_axis',(0.408248290463806,0.408248290463692,-0.81649658092784)) ;
#45278=DIRECTION('ref_axis',(-0.577350269189777,-0.57735026918955,-0.57735026918955)) ;
#45279=DIRECTION('center_axis',(-0.408248290463711,-0.816496580927764,0.408248290463939)) ;
#45280=DIRECTION('ref_axis',(0.57735026918955,-0.57735026918955,-0.577350269189777)) ;
#45281=DIRECTION('center_axis',(1.42108547152028E-13,2.17161023787773E-15,
1.)) ;
#45282=DIRECTION('ref_axis',(1.,0.,-1.515824502955E-13)) ;
#45283=DIRECTION('center_axis',(-1.42108547152028E-13,-2.17161023787773E-15,
-1.)) ;
#45284=DIRECTION('ref_axis',(-1.,0.,1.51582450295488E-13)) ;
#45285=DIRECTION('center_axis',(2.9073965457371E-15,-1.,2.17161023787728E-15)) ;
#45286=DIRECTION('ref_axis',(0.,0.,-1.)) ;
#45287=DIRECTION('center_axis',(-2.9073965457371E-15,1.,-2.17161023787728E-15)) ;
#45288=DIRECTION('ref_axis',(-1.49322507795023E-13,-2.17161023787771E-15,
-1.)) ;
#45289=DIRECTION('center_axis',(-1.,-2.9073965457371E-15,9.03687443371611E-30)) ;
#45290=DIRECTION('ref_axis',(0.,3.108235939458E-15,1.)) ;
#45291=DIRECTION('center_axis',(2.9073965457371E-15,-1.,2.17161023787728E-15)) ;
#45292=DIRECTION('ref_axis',(-1.49322507795023E-13,-2.17161023787771E-15,
-1.)) ;
#45293=DIRECTION('center_axis',(2.90739654573709E-15,-1.,2.17161023787725E-15)) ;
#45294=DIRECTION('ref_axis',(-1.48506207331423E-13,-2.17161023787768E-15,
-1.)) ;
#45295=DIRECTION('center_axis',(2.90739654573709E-15,-1.,2.17161023787725E-15)) ;
#45296=DIRECTION('ref_axis',(-9.93363673616178E-14,-2.17161023787754E-15,
-1.)) ;
#45297=DIRECTION('center_axis',(-2.9073965457371E-15,1.,-2.17161023787728E-15)) ;
#45298=DIRECTION('ref_axis',(-1.58279632150758E-13,-2.17161023787774E-15,
-1.)) ;
#45299=DIRECTION('center_axis',(-2.90739654573709E-15,1.,-2.17161023787725E-15)) ;
#45300=DIRECTION('ref_axis',(-9.93363673616178E-14,-2.17161023787754E-15,
-1.)) ;
#45301=DIRECTION('center_axis',(-2.90739654573709E-15,1.,-2.17161023787725E-15)) ;
#45302=DIRECTION('ref_axis',(-9.93363673616178E-14,-2.17161023787754E-15,
-1.)) ;
#45303=DIRECTION('',(2.9073965457371E-15,-1.,2.17161023787728E-15)) ;
#45304=DIRECTION('center_axis',(-2.90739654573709E-15,1.,-2.17161023787725E-15)) ;
#45305=DIRECTION('ref_axis',(0.,0.,1.)) ;
#45306=DIRECTION('center_axis',(1.,2.90739654573709E-15,-8.30985315988538E-30)) ;
#45307=DIRECTION('ref_axis',(0.,-2.85817673274378E-15,-1.)) ;
#45308=DIRECTION('center_axis',(2.9073965457371E-15,-1.,2.17161023787728E-15)) ;
#45309=DIRECTION('ref_axis',(1.48422940604576E-13,2.17161023787771E-15,
1.)) ;
#78787=CARTESIAN_POINT('',(0.,0.,0.)) ;
#78788=CARTESIAN_POINT('Origin',(130.842036869422,-80.5295274127545,-200.900005310181)) ;
#78789=CARTESIAN_POINT('',(130.842036869422,-75.5685899127545,-202.652605310181)) ;
#78790=CARTESIAN_POINT('',(130.842036869422,-75.4693711627547,-202.652605310181)) ;
#78791=CARTESIAN_POINT('',(130.842036869422,-80.5295274127545,-202.652605310181)) ;
#78792=CARTESIAN_POINT('',(129.538783258268,-75.178136333852,-199.72819611709)) ;
#78793=CARTESIAN_POINT('Ctrl Pts',(130.842036869422,-75.4693711627547,-202.652605310181)) ;
#78794=CARTESIAN_POINT('Ctrl Pts',(130.711623674148,-75.4604591013659,-202.652605310181)) ;
#78795=CARTESIAN_POINT('Ctrl Pts',(130.581350458606,-75.45114469441,-202.638053305016)) ;
#78796=CARTESIAN_POINT('Ctrl Pts',(130.229646191826,-75.424847544527,-202.558116804753)) ;
#78797=CARTESIAN_POINT('Ctrl Pts',(130.017854402449,-75.4077012196374,-202.463682049367)) ;
#78798=CARTESIAN_POINT('Ctrl Pts',(129.645404195784,-75.3747957460244,-202.200371817811)) ;
#78799=CARTESIAN_POINT('Ctrl Pts',(129.487601874771,-75.3597717165059,-202.035077120023)) ;
#78800=CARTESIAN_POINT('Ctrl Pts',(129.241759961654,-75.3265456678467,-201.650700216346)) ;
#78801=CARTESIAN_POINT('Ctrl Pts',(129.157209481383,-75.309384599292,-201.434598477145)) ;
#78802=CARTESIAN_POINT('Ctrl Pts',(129.076967738613,-75.2764311561231,-200.985616864913)) ;
#78803=CARTESIAN_POINT('Ctrl Pts',(129.080663347727,-75.261430802899,-200.757312650326)) ;
#78804=CARTESIAN_POINT('Ctrl Pts',(129.159604564136,-75.2337894460306,-200.385525890022)) ;
#78805=CARTESIAN_POINT('Ctrl Pts',(129.2112220981,-75.222378340329,-200.239924020435)) ;
#78806=CARTESIAN_POINT('Ctrl Pts',(129.350395585309,-75.1998143561719,-199.967385188184)) ;
#78807=CARTESIAN_POINT('Ctrl Pts',(129.436986777276,-75.1887546024267,-199.841411333558)) ;
#78808=CARTESIAN_POINT('Ctrl Pts',(129.538783258269,-75.1781363338561,-199.728196117089)) ;
#78809=CARTESIAN_POINT('',(130.749091630179,-75.1781363338479,-199.14987161743)) ;
#78810=CARTESIAN_POINT('Origin',(130.842036869422,-75.1781363338479,-200.900005310181)) ;
#78811=CARTESIAN_POINT('Ctrl Pts',(130.749091630179,-75.1781363338479,-199.14987161743)) ;
#78812=CARTESIAN_POINT('Ctrl Pts',(130.583254486741,-75.1897184635544,-199.158678814867)) ;
#78813=CARTESIAN_POINT('Ctrl Pts',(130.419542420933,-75.2018212127873,-199.191008850173)) ;
#78814=CARTESIAN_POINT('Ctrl Pts',(130.104891265179,-75.2264421770496,-199.301183187997)) ;
#78815=CARTESIAN_POINT('Ctrl Pts',(129.955658398848,-75.238838371062,-199.378835920221)) ;
#78816=CARTESIAN_POINT('Ctrl Pts',(129.636699798695,-75.2671190344011,-199.607901016349)) ;
#78817=CARTESIAN_POINT('Ctrl Pts',(129.480768268154,-75.2820839842016,-199.77336511249)) ;
#78818=CARTESIAN_POINT('Ctrl Pts',(129.237096602546,-75.3153352420707,-200.15900985697)) ;
#78819=CARTESIAN_POINT('Ctrl Pts',(129.153543957048,-75.3325729348049,-200.376646180286)) ;
#78820=CARTESIAN_POINT('Ctrl Pts',(129.076532892538,-75.3654879406052,-200.826403516307)) ;
#78821=CARTESIAN_POINT('Ctrl Pts',(129.081706866303,-75.3804449144316,-201.053820825158)) ;
#78822=CARTESIAN_POINT('Ctrl Pts',(129.179055347663,-75.4136531396854,-201.499444906297)) ;
#78823=CARTESIAN_POINT('Ctrl Pts',(129.272321466205,-75.4308815313005,-201.712921670936)) ;
#78824=CARTESIAN_POINT('Ctrl Pts',(129.533230085197,-75.4638459969484,-202.08722990841)) ;
#78825=CARTESIAN_POINT('Ctrl Pts',(129.696689211027,-75.4787997245241,-202.245611390901)) ;
#78826=CARTESIAN_POINT('Ctrl Pts',(130.078901162208,-75.5119638302814,-202.494491642853)) ;
#78827=CARTESIAN_POINT('Ctrl Pts',(130.295049123513,-75.5291820177327,-202.580948429471)) ;
#78828=CARTESIAN_POINT('Ctrl Pts',(130.627614758952,-75.553658530876,-202.64277021834)) ;
#78829=CARTESIAN_POINT('Ctrl Pts',(130.73482723915,-75.5612635160318,-202.652605310181)) ;
#78830=CARTESIAN_POINT('Ctrl Pts',(130.842036869422,-75.5685899127545,-202.652605310181)) ;
#78831=CARTESIAN_POINT('Origin',(130.842036869422,-80.5295274127545,-200.900005310181)) ;
#78832=CARTESIAN_POINT('',(130.842036869422,-76.3623399127545,-202.652605310181)) ;
#78833=CARTESIAN_POINT('',(130.842036869422,-76.2631211627547,-202.652605310181)) ;
#78834=CARTESIAN_POINT('',(130.842036869422,-80.5295274127545,-202.652605310181)) ;
#78835=CARTESIAN_POINT('Ctrl Pts',(130.842036869423,-76.2631211627547,-202.652605310181)) ;
#78836=CARTESIAN_POINT('Ctrl Pts',(130.680530862958,-76.2520843083839,-202.652605310181)) ;
#78837=CARTESIAN_POINT('Ctrl Pts',(130.519524607284,-76.240449888059,-202.630287995016)) ;
#78838=CARTESIAN_POINT('Ctrl Pts',(130.143742521215,-76.2117513287222,-202.523643499451)) ;
#78839=CARTESIAN_POINT('Ctrl Pts',(129.938218404822,-76.1947406166118,-202.418868171205)) ;
#78840=CARTESIAN_POINT('Ctrl Pts',(129.579230443517,-76.1622165224726,-202.136530578372)) ;
#78841=CARTESIAN_POINT('Ctrl Pts',(129.429150307446,-76.1468603032157,-201.961809848165)) ;
#78842=CARTESIAN_POINT('Ctrl Pts',(129.204152299825,-76.1133229218017,-201.564243279102)) ;
#78843=CARTESIAN_POINT('Ctrl Pts',(129.131552208418,-76.09629426262,-201.345129117699)) ;
#78844=CARTESIAN_POINT('Ctrl Pts',(129.074692618702,-76.063724019615,-200.89206979759)) ;
#78845=CARTESIAN_POINT('Ctrl Pts',(129.090700039042,-76.0484202449793,-200.662540463456)) ;
#78846=CARTESIAN_POINT('Ctrl Pts',(129.209927517257,-76.0149164496177,-200.22165378263)) ;
#78847=CARTESIAN_POINT('Ctrl Pts',(129.312316492737,-75.997869967443,-200.01461777116)) ;
#78848=CARTESIAN_POINT('Ctrl Pts',(129.590225701037,-75.9652528792995,-199.652434700344)) ;
#78849=CARTESIAN_POINT('Ctrl Pts',(129.762719252203,-75.9499991490224,-199.500527579452)) ;
#78850=CARTESIAN_POINT('Ctrl Pts',(130.157227417958,-75.9165305241439,-199.270574963972)) ;
#78851=CARTESIAN_POINT('Ctrl Pts',(130.375689145037,-75.8994664234005,-199.195147677286)) ;
#78852=CARTESIAN_POINT('Ctrl Pts',(130.827837753823,-75.8668019164062,-199.132759277728)) ;
#78853=CARTESIAN_POINT('Ctrl Pts',(131.057076696894,-75.8515954494147,-199.145833643124)) ;
#78854=CARTESIAN_POINT('Ctrl Pts',(131.499315712216,-75.8181635650319,-199.259255825996)) ;
#78855=CARTESIAN_POINT('Ctrl Pts',(131.707911547695,-75.8010821313174,-199.359113821189)) ;
#78856=CARTESIAN_POINT('Ctrl Pts',(132.073423739357,-75.7683697617454,-199.632351923101)) ;
#78857=CARTESIAN_POINT('Ctrl Pts',(132.227237627881,-75.7532074074886,-199.80251847069)) ;
#78858=CARTESIAN_POINT('Ctrl Pts',(132.462347492692,-75.7198138065936,-200.193792582609)) ;
#78859=CARTESIAN_POINT('Ctrl Pts',(132.540726942963,-75.7027154063227,-200.41153340003)) ;
#78860=CARTESIAN_POINT('Ctrl Pts',(132.60888938881,-75.6699548665787,-200.862695600096)) ;
#78861=CARTESIAN_POINT('Ctrl Pts',(132.598863206262,-75.6548331230282,-201.091631358305)) ;
#78862=CARTESIAN_POINT('Ctrl Pts',(132.491490612412,-75.6214793083452,-201.535233775242)) ;
#78863=CARTESIAN_POINT('Ctrl Pts',(132.394291290212,-75.6043643871491,-201.74542090273)) ;
#78864=CARTESIAN_POINT('Ctrl Pts',(132.125933368952,-75.5715555104706,-202.114366752397)) ;
#78865=CARTESIAN_POINT('Ctrl Pts',(131.958174035764,-75.556470548808,-202.270151684134)) ;
#78866=CARTESIAN_POINT('Ctrl Pts',(131.570286632123,-75.5231579691041,-202.51057546937)) ;
#78867=CARTESIAN_POINT('Ctrl Pts',(131.353333758772,-75.5060270489619,-202.592006046919)) ;
#78868=CARTESIAN_POINT('Ctrl Pts',(131.032490736109,-75.4826057764187,-202.644849186622)) ;
#78869=CARTESIAN_POINT('Ctrl Pts',(130.937241579496,-75.4758771778776,-202.652605310181)) ;
#78870=CARTESIAN_POINT('Ctrl Pts',(130.842036869422,-75.4693711627547,-202.652605310181)) ;
#78871=CARTESIAN_POINT('Ctrl Pts',(130.842036869422,-75.5685899127545,-202.652605310181)) ;
#78872=CARTESIAN_POINT('Ctrl Pts',(130.959477744642,-75.5766154832293,-202.652605310181)) ;
#78873=CARTESIAN_POINT('Ctrl Pts',(131.076869305746,-75.5849717373026,-202.640803865211)) ;
#78874=CARTESIAN_POINT('Ctrl Pts',(131.41821150113,-75.6102698116508,-202.571146452148)) ;
#78875=CARTESIAN_POINT('Ctrl Pts',(131.632673993324,-75.6274769034568,-202.481012570103)) ;
#78876=CARTESIAN_POINT('Ctrl Pts',(132.010645484719,-75.6605387180287,-202.225508685628)) ;
#78877=CARTESIAN_POINT('Ctrl Pts',(132.171518155561,-75.6755006059372,-202.064086384525)) ;
#78878=CARTESIAN_POINT('Ctrl Pts',(132.425641905301,-75.7085736307167,-201.685379179858)) ;
#78879=CARTESIAN_POINT('Ctrl Pts',(132.515009981141,-75.725768754759,-201.470774608662)) ;
#78880=CARTESIAN_POINT('Ctrl Pts',(132.604827890813,-75.7588782129851,-201.023476553771)) ;
#78881=CARTESIAN_POINT('Ctrl Pts',(132.606049116628,-75.7738515041829,-200.795418974851)) ;
#78882=CARTESIAN_POINT('Ctrl Pts',(132.521055612484,-75.8068778545833,-200.347338730559)) ;
#78883=CARTESIAN_POINT('Ctrl Pts',(132.43408062645,-75.8240601663205,-200.131930395886)) ;
#78884=CARTESIAN_POINT('Ctrl Pts',(132.184038144773,-75.8572163801247,-199.750315341626)) ;
#78885=CARTESIAN_POINT('Ctrl Pts',(132.024665724764,-75.8722059667016,-199.586938734511)) ;
#78886=CARTESIAN_POINT('Ctrl Pts',(131.649496464221,-75.9051850367174,-199.32759286598)) ;
#78887=CARTESIAN_POINT('Ctrl Pts',(131.436473815438,-75.9223537365705,-199.235339205358)) ;
#78888=CARTESIAN_POINT('Ctrl Pts',(130.990483732311,-75.9555556730147,-199.139096502026)) ;
#78889=CARTESIAN_POINT('Ctrl Pts',(130.762105493726,-75.9705663911608,-199.134658928056)) ;
#78890=CARTESIAN_POINT('Ctrl Pts',(130.312859003515,-76.0034976947888,-199.213479053113)) ;
#78891=CARTESIAN_POINT('Ctrl Pts',(130.0965551513,-76.0206520317887,-199.297303777041)) ;
#78892=CARTESIAN_POINT('Ctrl Pts',(129.711357293294,-76.0538985433324,-199.541886643868)) ;
#78893=CARTESIAN_POINT('Ctrl Pts',(129.545488935552,-76.0689350880305,-199.699219419944)) ;
#78894=CARTESIAN_POINT('Ctrl Pts',(129.280999183371,-76.1018182804073,-200.070855004335)) ;
#78895=CARTESIAN_POINT('Ctrl Pts',(129.185917130932,-76.1189575601195,-200.28227558004)) ;
#78896=CARTESIAN_POINT('Ctrl Pts',(129.083328343325,-76.1522473970365,-200.726923306207)) ;
#78897=CARTESIAN_POINT('Ctrl Pts',(129.075707100053,-76.1673142726,-200.955619260857)) ;
#78898=CARTESIAN_POINT('Ctrl Pts',(129.148444787698,-76.2001491530251,-201.405974185939)) ;
#78899=CARTESIAN_POINT('Ctrl Pts',(129.22916264484,-76.2172727445578,-201.623115035738)) ;
#78900=CARTESIAN_POINT('Ctrl Pts',(129.468346539637,-76.2506045681308,-202.01179762083)) ;
#78901=CARTESIAN_POINT('Ctrl Pts',(129.623670940997,-76.2657060428676,-202.180119503146)) ;
#78902=CARTESIAN_POINT('Ctrl Pts',(129.991815319861,-76.2984925560701,-202.449622289195)) ;
#78903=CARTESIAN_POINT('Ctrl Pts',(130.201632658185,-76.3155998980288,-202.547446602108)) ;
#78904=CARTESIAN_POINT('Ctrl Pts',(130.561330991605,-76.3426794053451,-202.635722841674)) ;
#78905=CARTESIAN_POINT('Ctrl Pts',(130.701567106792,-76.3527406145762,-202.652605310181)) ;
#78906=CARTESIAN_POINT('Ctrl Pts',(130.842036869422,-76.3623399127545,-202.652605310181)) ;
#78907=CARTESIAN_POINT('Origin',(130.842036869422,-80.5295274127545,-200.900005310181)) ;
#78908=CARTESIAN_POINT('',(130.842036869422,-77.1560899127545,-202.652605310181)) ;
#78909=CARTESIAN_POINT('',(130.842036869422,-77.0568711627547,-202.652605310181)) ;
#78910=CARTESIAN_POINT('',(130.842036869422,-80.5295274127545,-202.652605310181)) ;
#78911=CARTESIAN_POINT('Ctrl Pts',(130.842036869423,-77.0568711627547,-202.652605310181)) ;
#78912=CARTESIAN_POINT('Ctrl Pts',(130.660862359968,-77.0444902196534,-202.652605310181)) ;
#78913=CARTESIAN_POINT('Ctrl Pts',(130.480554613838,-77.0313735225802,-202.62452004209)) ;
#78914=CARTESIAN_POINT('Ctrl Pts',(130.085697399116,-77.000810765977,-202.498068619796)) ;
#78915=CARTESIAN_POINT('Ctrl Pts',(129.880224218456,-76.983526713373,-202.383513748854)) ;
#78916=CARTESIAN_POINT('Ctrl Pts',(129.532288465508,-76.9513296806648,-202.086048190946)) ;
#78917=CARTESIAN_POINT('Ctrl Pts',(129.391113123426,-76.9358875977997,-201.908456427025)) ;
#78918=CARTESIAN_POINT('Ctrl Pts',(129.179864391872,-76.9021655650029,-201.502492655479)) ;
#78919=CARTESIAN_POINT('Ctrl Pts',(129.114605521132,-76.8848805664655,-201.276586560807)) ;
#78920=CARTESIAN_POINT('Ctrl Pts',(129.07687057682,-76.8526447943419,-200.82049997823)) ;
#78921=CARTESIAN_POINT('Ctrl Pts',(129.101600837785,-76.8372461483228,-200.594999757667)) ;
#78922=CARTESIAN_POINT('Ctrl Pts',(129.237269162886,-76.8035468524068,-200.158062273154)) ;
#78923=CARTESIAN_POINT('Ctrl Pts',(129.349858198285,-76.786261223496,-199.951751750124)) ;
#78924=CARTESIAN_POINT('Ctrl Pts',(129.643953164324,-76.7539853070896,-199.601265520593)) ;
#78925=CARTESIAN_POINT('Ctrl Pts',(129.820211604413,-76.7386299006385,-199.458473588984)) ;
#78926=CARTESIAN_POINT('Ctrl Pts',(130.223983964321,-76.7049546806224,-199.243588123652)) ;
#78927=CARTESIAN_POINT('Ctrl Pts',(130.449047202455,-76.6876687850883,-199.176262728122)) ;
#78928=CARTESIAN_POINT('Ctrl Pts',(130.909073090394,-76.6550281376619,-199.133734673547)) ;
#78929=CARTESIAN_POINT('Ctrl Pts',(131.139374153986,-76.6393870344989,-199.157648888211)) ;
#78930=CARTESIAN_POINT('Ctrl Pts',(131.576419558745,-76.6057052246166,-199.292438924183)) ;
#78931=CARTESIAN_POINT('Ctrl Pts',(131.77911781247,-76.5887660217225,-199.401510210809)) ;
#78932=CARTESIAN_POINT('Ctrl Pts',(132.132208948266,-76.5564174246657,-199.691884038837)) ;
#78933=CARTESIAN_POINT('Ctrl Pts',(132.278922193298,-76.5408350866697,-199.870700004851)) ;
#78934=CARTESIAN_POINT('Ctrl Pts',(132.494762704611,-76.5071791018237,-200.273795297035)) ;
#78935=CARTESIAN_POINT('Ctrl Pts',(132.562162396617,-76.490222206561,-200.494013388806)) ;
#78936=CARTESIAN_POINT('Ctrl Pts',(132.608849707334,-76.4578312887575,-200.948662078778)) ;
#78937=CARTESIAN_POINT('Ctrl Pts',(132.587407092316,-76.4423071791597,-201.178724080473)) ;
#78938=CARTESIAN_POINT('Ctrl Pts',(132.457467252682,-76.408678519364,-201.617000739225)) ;
#78939=CARTESIAN_POINT('Ctrl Pts',(132.350462124597,-76.3917037628473,-201.821075091975)) ;
#78940=CARTESIAN_POINT('Ctrl Pts',(132.063964068573,-76.3592694308844,-202.177026212854)) ;
#78941=CARTESIAN_POINT('Ctrl Pts',(131.887131888661,-76.3438026630912,-202.325371835702)) ;
#78942=CARTESIAN_POINT('Ctrl Pts',(131.486699375041,-76.3102028625554,-202.545655983835)) ;
#78943=CARTESIAN_POINT('Ctrl Pts',(131.267000568947,-76.293210143172,-202.615574936906)) ;
#78944=CARTESIAN_POINT('Ctrl Pts',(130.974192440467,-76.2722579522,-202.648872584618)) ;
#78945=CARTESIAN_POINT('Ctrl Pts',(130.908080100251,-76.2676343665469,-202.652605310181)) ;
#78946=CARTESIAN_POINT('Ctrl Pts',(130.842036869423,-76.2631211627547,-202.652605310181)) ;
#78947=CARTESIAN_POINT('Ctrl Pts',(130.842036869422,-76.3623399127545,-202.652605310181)) ;
#78948=CARTESIAN_POINT('Ctrl Pts',(130.927732020547,-76.3681960720637,-202.652605310181)) ;
#78949=CARTESIAN_POINT('Ctrl Pts',(131.013489712243,-76.3742343886244,-202.646321045107)) ;
#78950=CARTESIAN_POINT('Ctrl Pts',(131.325323374,-76.396850595793,-202.600168733674)) ;
#78951=CARTESIAN_POINT('Ctrl Pts',(131.543236919714,-76.4139412010658,-202.52248166809)) ;
#78952=CARTESIAN_POINT('Ctrl Pts',(131.935273278315,-76.4473526944659,-202.288579923138)) ;
#78953=CARTESIAN_POINT('Ctrl Pts',(132.105985750161,-76.4625350327593,-202.135213217096)) ;
#78954=CARTESIAN_POINT('Ctrl Pts',(132.380323796131,-76.4952252232096,-201.770481191732)) ;
#78955=CARTESIAN_POINT('Ctrl Pts',(132.480779023794,-76.5122986825163,-201.562249430233)) ;
#78956=CARTESIAN_POINT('Ctrl Pts',(132.595566916625,-76.545747750087,-201.120324663123)) ;
#78957=CARTESIAN_POINT('Ctrl Pts',(132.609330561055,-76.56097570292,-200.891017337064)) ;
#78958=CARTESIAN_POINT('Ctrl Pts',(132.548243878357,-76.5936182194001,-200.438651334102)) ;
#78959=CARTESIAN_POINT('Ctrl Pts',(132.473482223509,-76.6106742035755,-200.22003266576)) ;
#78960=CARTESIAN_POINT('Ctrl Pts',(132.244694692041,-76.6441592882175,-199.824801045146)) ;
#78961=CARTESIAN_POINT('Ctrl Pts',(132.093217587578,-76.6594358371184,-199.651783035504)) ;
#78962=CARTESIAN_POINT('Ctrl Pts',(131.729342273886,-76.6922515818963,-199.370941121313)) ;
#78963=CARTESIAN_POINT('Ctrl Pts',(131.519544627757,-76.7095273473052,-199.267119203586)) ;
#78964=CARTESIAN_POINT('Ctrl Pts',(131.078444100614,-76.7430165317484,-199.148924170579)) ;
#78965=CARTESIAN_POINT('Ctrl Pts',(130.852083649157,-76.7581224862258,-199.133067137667)) ;
#78966=CARTESIAN_POINT('Ctrl Pts',(130.398646477582,-76.7906817392251,-199.188626258328)) ;
#78967=CARTESIAN_POINT('Ctrl Pts',(130.176299310019,-76.8079607520649,-199.262265676444)) ;
#78968=CARTESIAN_POINT('Ctrl Pts',(129.779379757525,-76.841483184078,-199.488297587811)) ;
#78969=CARTESIAN_POINT('Ctrl Pts',(129.607247921277,-76.8566236548969,-199.636101837318)) ;
#78970=CARTESIAN_POINT('Ctrl Pts',(129.323693542478,-76.8891354594,-199.994405950988)) ;
#78971=CARTESIAN_POINT('Ctrl Pts',(129.217251752075,-76.9064170276745,-200.203203325608)) ;
#78972=CARTESIAN_POINT('Ctrl Pts',(129.093852777237,-76.9399712233906,-200.643099641315)) ;
#78973=CARTESIAN_POINT('Ctrl Pts',(129.075346457736,-76.9551485249676,-200.869201516679)) ;
#78974=CARTESIAN_POINT('Ctrl Pts',(129.125582008963,-76.9876137783497,-201.323468254862)) ;
#78975=CARTESIAN_POINT('Ctrl Pts',(129.196731061098,-77.0048972601188,-201.54691236114)) ;
#78976=CARTESIAN_POINT('Ctrl Pts',(129.418359724146,-77.0384817382174,-201.946563740064)) ;
#78977=CARTESIAN_POINT('Ctrl Pts',(129.564173231869,-77.0536978199423,-202.120333179967)) ;
#78978=CARTESIAN_POINT('Ctrl Pts',(129.919389102757,-77.0861175319037,-202.408089791066)) ;
#78979=CARTESIAN_POINT('Ctrl Pts',(130.127218863722,-77.1034023371828,-202.516981964381)) ;
#78980=CARTESIAN_POINT('Ctrl Pts',(130.510261782241,-77.1327485220846,-202.628976575734)) ;
#78981=CARTESIAN_POINT('Ctrl Pts',(130.675853792087,-77.1447334408586,-202.652605310181)) ;
#78982=CARTESIAN_POINT('Ctrl Pts',(130.842036869423,-77.1560899127545,-202.652605310181)) ;
#78983=CARTESIAN_POINT('Origin',(130.842036869422,-80.5295274127545,-200.900005310181)) ;
#78984=CARTESIAN_POINT('',(130.842036869422,-77.9498399127545,-202.652605310181)) ;
#78985=CARTESIAN_POINT('',(130.842036869422,-77.8506211627547,-202.652605310181)) ;
#78986=CARTESIAN_POINT('',(130.842036869422,-80.5295274127545,-202.652605310181)) ;
#78987=CARTESIAN_POINT('',(132.582591005309,-78.1626363340786,-200.694875936254)) ;
#78988=CARTESIAN_POINT('Ctrl Pts',(130.842036869422,-77.9498399127545,-202.652605310181)) ;
#78989=CARTESIAN_POINT('Ctrl Pts',(130.878973335089,-77.9523640442185,-202.652605310181)) ;
#78990=CARTESIAN_POINT('Ctrl Pts',(130.915944065332,-77.9549235685973,-202.651437671282)) ;
#78991=CARTESIAN_POINT('Ctrl Pts',(131.185735954615,-77.9738443881084,-202.63433819772)) ;
#78992=CARTESIAN_POINT('Ctrl Pts',(131.413270636545,-77.9911230002116,-202.57323670437)) ;
#78993=CARTESIAN_POINT('Ctrl Pts',(131.823569757904,-78.0249345862475,-202.369290696316)) ;
#78994=CARTESIAN_POINT('Ctrl Pts',(132.00382073611,-78.0405744142742,-202.231335498657)) ;
#78995=CARTESIAN_POINT('Ctrl Pts',(132.307955670742,-78.0726103610347,-201.88851951691)) ;
#78996=CARTESIAN_POINT('Ctrl Pts',(132.426398965465,-78.0898871114286,-201.684763829815)) ;
#78997=CARTESIAN_POINT('Ctrl Pts',(132.543724247562,-78.1168050533483,-201.339462244637)) ;
#78998=CARTESIAN_POINT('Ctrl Pts',(132.571871931176,-78.1264000599994,-201.210714433672)) ;
#78999=CARTESIAN_POINT('Ctrl Pts',(132.598595450617,-78.1448420342225,-200.951916059058)) ;
#79000=CARTESIAN_POINT('Ctrl Pts',(132.597664960051,-78.1534690027399,-200.822780749546)) ;
#79001=CARTESIAN_POINT('Ctrl Pts',(132.582591005311,-78.1626363343082,-200.69487593627)) ;
#79002=CARTESIAN_POINT('',(131.927746207111,-78.1626363319089,-199.524199363257)) ;
#79003=CARTESIAN_POINT('Origin',(130.842036869422,-78.162636333848,-200.900005310181)) ;
#79004=CARTESIAN_POINT('Ctrl Pts',(131.92774620522,-78.1626363275436,-199.524199365231)) ;
#79005=CARTESIAN_POINT('Ctrl Pts',(132.032870635821,-78.1531041953848,-199.607157704045)) ;
#79006=CARTESIAN_POINT('Ctrl Pts',(132.128113721767,-78.1441417575876,-199.70186258093)) ;
#79007=CARTESIAN_POINT('Ctrl Pts',(132.296967822098,-78.1249092162616,-199.913357175936)) ;
#79008=CARTESIAN_POINT('Ctrl Pts',(132.369466681103,-78.1148993723112,-200.029804582434)) ;
#79009=CARTESIAN_POINT('Ctrl Pts',(132.527258877092,-78.0875293201199,-200.364960104891)) ;
#79010=CARTESIAN_POINT('Ctrl Pts',(132.583533118867,-78.0702656353602,-200.594275863051)) ;
#79011=CARTESIAN_POINT('Ctrl Pts',(132.602412482054,-78.038398844302,-201.052773258879)) ;
#79012=CARTESIAN_POINT('Ctrl Pts',(132.568271995862,-78.0225237872543,-201.277378390298)) ;
#79013=CARTESIAN_POINT('Ctrl Pts',(132.413961440197,-77.9886262611793,-201.709494778747)) ;
#79014=CARTESIAN_POINT('Ctrl Pts',(132.29212573684,-77.9713604947043,-201.911684552793)) ;
#79015=CARTESIAN_POINT('Ctrl Pts',(131.982167398814,-77.9394706930005,-202.249949812049)) ;
#79016=CARTESIAN_POINT('Ctrl Pts',(131.799570632373,-77.9236291961254,-202.385068504199)) ;
#79017=CARTESIAN_POINT('Ctrl Pts',(131.385487786747,-77.889742898508,-202.582519204571)) ;
#79018=CARTESIAN_POINT('Ctrl Pts',(131.156575821523,-77.8724750331792,-202.639915979879)) ;
#79019=CARTESIAN_POINT('Ctrl Pts',(130.896087871841,-77.8543325329972,-202.651980685353)) ;
#79020=CARTESIAN_POINT('Ctrl Pts',(130.869052052766,-77.8524673024178,-202.652605310181)) ;
#79021=CARTESIAN_POINT('Ctrl Pts',(130.842036869422,-77.8506211627547,-202.652605310181)) ;
#79022=CARTESIAN_POINT('Origin',(130.842036869422,-75.6433781549656,-200.900005310181)) ;
#79023=CARTESIAN_POINT('',(130.842036869422,-75.7204074847575,-199.400005310181)) ;
#79024=CARTESIAN_POINT('',(130.842036869422,-75.3175535907516,-199.400005310181)) ;
#79025=CARTESIAN_POINT('',(130.842036869422,-75.6433781549656,-199.400005310181)) ;
#79026=CARTESIAN_POINT('',(132.182528457453,-75.1781363338479,-200.226891425003)) ;
#79027=CARTESIAN_POINT('Ctrl Pts',(130.842036869422,-75.3175535907516,-199.400005310181)) ;
#79028=CARTESIAN_POINT('Ctrl Pts',(130.923497640682,-75.3110493486307,-199.400005310181)) ;
#79029=CARTESIAN_POINT('Ctrl Pts',(131.00499096693,-75.304323094454,-199.40663952094)) ;
#79030=CARTESIAN_POINT('Ctrl Pts',(131.281007794349,-75.2807814784863,-199.452085443423)) ;
#79031=CARTESIAN_POINT('Ctrl Pts',(131.467996781686,-75.2635202774295,-199.522567574949)) ;
#79032=CARTESIAN_POINT('Ctrl Pts',(131.751702866556,-75.2350150020201,-199.699532289036)) ;
#79033=CARTESIAN_POINT('Ctrl Pts',(131.857062122586,-75.2240076020635,-199.787200645029)) ;
#79034=CARTESIAN_POINT('Ctrl Pts',(132.042145181341,-75.2017219599688,-199.989647742754)) ;
#79035=CARTESIAN_POINT('Ctrl Pts',(132.120680804841,-75.1900161952267,-200.103723176819)) ;
#79036=CARTESIAN_POINT('Ctrl Pts',(132.182528457453,-75.1781363338479,-200.226891425003)) ;
#79037=CARTESIAN_POINT('',(129.471900051694,-75.1781363338479,-201.5105174728)) ;
#79038=CARTESIAN_POINT('Origin',(130.842036869422,-75.1781363338479,-200.900005310181)) ;
#79039=CARTESIAN_POINT('Ctrl Pts',(129.471900051693,-75.1781363338479,-201.510517472799)) ;
#79040=CARTESIAN_POINT('Ctrl Pts',(129.523145180104,-75.1890138594523,-201.62552392388)) ;
#79041=CARTESIAN_POINT('Ctrl Pts',(129.588668562329,-75.1998125962201,-201.733629357294)) ;
#79042=CARTESIAN_POINT('Ctrl Pts',(129.743608209588,-75.2205300543474,-201.928921932756)) ;
#79043=CARTESIAN_POINT('Ctrl Pts',(129.831872765876,-75.2301658928566,-202.015704331718)) ;
#79044=CARTESIAN_POINT('Ctrl Pts',(130.085406381744,-75.256833387257,-202.209944277907)) ;
#79045=CARTESIAN_POINT('Ctrl Pts',(130.262879102329,-75.2738994471159,-202.297500377412)) ;
#79046=CARTESIAN_POINT('Ctrl Pts',(130.640660017268,-75.3074266408475,-202.399192190453)) ;
#79047=CARTESIAN_POINT('Ctrl Pts',(130.837245993353,-75.3227318075518,-202.41264856471)) ;
#79048=CARTESIAN_POINT('Ctrl Pts',(131.225288586058,-75.3553440832905,-202.363394295449)) ;
#79049=CARTESIAN_POINT('Ctrl Pts',(131.412936549342,-75.3723944027559,-202.30087933489)) ;
#79050=CARTESIAN_POINT('Ctrl Pts',(131.75312498777,-75.4059516029996,-202.107523971697)) ;
#79051=CARTESIAN_POINT('Ctrl Pts',(131.902486230923,-75.4213026058212,-201.978721156193)) ;
#79052=CARTESIAN_POINT('Ctrl Pts',(132.143713490584,-75.453873769828,-201.670711273436)) ;
#79053=CARTESIAN_POINT('Ctrl Pts',(132.233094454037,-75.4709082764385,-201.494389617103)) ;
#79054=CARTESIAN_POINT('Ctrl Pts',(132.338999307863,-75.5044941579365,-201.117618780385)) ;
#79055=CARTESIAN_POINT('Ctrl Pts',(132.354589568972,-75.5198925313956,-200.920824362433)) ;
#79056=CARTESIAN_POINT('Ctrl Pts',(132.309343323413,-75.5524233019008,-200.532142384087)) ;
#79057=CARTESIAN_POINT('Ctrl Pts',(132.248877081164,-75.5694419833218,-200.344042056749)) ;
#79058=CARTESIAN_POINT('Ctrl Pts',(132.059122564365,-75.6030552274161,-200.00166019157)) ;
#79059=CARTESIAN_POINT('Ctrl Pts',(131.931645903337,-75.6185022127119,-199.850686675688)) ;
#79060=CARTESIAN_POINT('Ctrl Pts',(131.625957549094,-75.6509933889424,-199.606273278445)) ;
#79061=CARTESIAN_POINT('Ctrl Pts',(131.450740290742,-75.6679962906386,-199.515181675565)) ;
#79062=CARTESIAN_POINT('Ctrl Pts',(131.125990033399,-75.6970664972799,-199.420224974047)) ;
#79063=CARTESIAN_POINT('Ctrl Pts',(130.98426630219,-75.7090511637559,-199.400005310181)) ;
#79064=CARTESIAN_POINT('Ctrl Pts',(130.842036869421,-75.7204074847575,-199.400005310181)) ;
#79065=CARTESIAN_POINT('Origin',(130.842036869422,-75.6433781549656,-200.900005310181)) ;
#79066=CARTESIAN_POINT('',(130.842036869422,-76.5141574847575,-199.400005310181)) ;
#79067=CARTESIAN_POINT('',(130.842036869422,-76.1113035907516,-199.400005310181)) ;
#79068=CARTESIAN_POINT('',(130.842036869422,-75.6433781549656,-199.400005310181)) ;
#79069=CARTESIAN_POINT('Ctrl Pts',(130.842036869422,-76.1113035907516,-199.400005310181)) ;
#79070=CARTESIAN_POINT('Ctrl Pts',(130.949133951451,-76.1027524152448,-199.400005310181)) ;
#79071=CARTESIAN_POINT('Ctrl Pts',(131.056137952684,-76.0938294801729,-199.411470631266)) ;
#79072=CARTESIAN_POINT('Ctrl Pts',(131.35367248696,-76.0679295416266,-199.476274975455)) ;
#79073=CARTESIAN_POINT('Ctrl Pts',(131.535967499815,-76.0507484264606,-199.555667869188)) ;
#79074=CARTESIAN_POINT('Ctrl Pts',(131.856884803169,-76.0177530719082,-199.778559777848)) ;
#79075=CARTESIAN_POINT('Ctrl Pts',(131.993103698459,-76.0027441261626,-199.918882943764)) ;
#79076=CARTESIAN_POINT('Ctrl Pts',(132.206435794837,-75.9695406232978,-200.246366953058)) ;
#79077=CARTESIAN_POINT('Ctrl Pts',(132.280411469569,-75.9523470991235,-200.431061265048)) ;
#79078=CARTESIAN_POINT('Ctrl Pts',(132.352103988871,-75.9193090849539,-200.815141685916)) ;
#79079=CARTESIAN_POINT('Ctrl Pts',(132.350440326257,-75.9043164329487,-201.010564209893)) ;
#79080=CARTESIAN_POINT('Ctrl Pts',(132.272196408425,-75.8711545191446,-201.393482702957)) ;
#79081=CARTESIAN_POINT('Ctrl Pts',(132.195018141393,-75.8539492166687,-201.576997972207)) ;
#79082=CARTESIAN_POINT('Ctrl Pts',(131.976138215843,-75.8208689999167,-201.900639928999)) ;
#79083=CARTESIAN_POINT('Ctrl Pts',(131.837740354137,-75.8058886898989,-202.038438444838)) ;
#79084=CARTESIAN_POINT('Ctrl Pts',(131.513051259311,-75.7727691594772,-202.255979052327)) ;
#79085=CARTESIAN_POINT('Ctrl Pts',(131.329077594801,-75.7555527454817,-202.33238662566)) ;
#79086=CARTESIAN_POINT('Ctrl Pts',(130.945923266647,-75.7224308342911,-202.408851659376)) ;
#79087=CARTESIAN_POINT('Ctrl Pts',(130.750746000305,-75.7074589752768,-202.409666134416)) ;
#79088=CARTESIAN_POINT('Ctrl Pts',(130.366844379053,-75.6743824609859,-202.336377856499)) ;
#79089=CARTESIAN_POINT('Ctrl Pts',(130.182132440041,-75.65715563652,-202.261437862205)) ;
#79090=CARTESIAN_POINT('Ctrl Pts',(129.85578178882,-75.6239926625053,-202.046595036644)) ;
#79091=CARTESIAN_POINT('Ctrl Pts',(129.716409296074,-75.6090253037173,-201.910119156804)) ;
#79092=CARTESIAN_POINT('Ctrl Pts',(129.494688502418,-75.5759923565716,-201.588245942602)) ;
#79093=CARTESIAN_POINT('Ctrl Pts',(129.415861126859,-75.5587558370719,-201.405022786578)) ;
#79094=CARTESIAN_POINT('Ctrl Pts',(129.334640315407,-75.5255525576802,-201.022819290159)) ;
#79095=CARTESIAN_POINT('Ctrl Pts',(129.331365796756,-75.5105857242824,-200.827887032132)) ;
#79096=CARTESIAN_POINT('Ctrl Pts',(129.399727674285,-75.4775968060397,-200.44304190406)) ;
#79097=CARTESIAN_POINT('Ctrl Pts',(129.472428123445,-75.460351321514,-200.257168611777)) ;
#79098=CARTESIAN_POINT('Ctrl Pts',(129.683247340528,-75.4271085811011,-199.928152312836)) ;
#79099=CARTESIAN_POINT('Ctrl Pts',(129.817824620494,-75.412138369452,-199.787224430205)) ;
#79100=CARTESIAN_POINT('Ctrl Pts',(130.136887807839,-75.3791938198857,-199.561392440293)) ;
#79101=CARTESIAN_POINT('Ctrl Pts',(130.319338815088,-75.3619401079321,-199.480181097861)) ;
#79102=CARTESIAN_POINT('Ctrl Pts',(130.620752245873,-75.3356272410693,-199.412255846619)) ;
#79103=CARTESIAN_POINT('Ctrl Pts',(130.731332038619,-75.3263928272623,-199.400005310181)) ;
#79104=CARTESIAN_POINT('Ctrl Pts',(130.842036869422,-75.3175535907516,-199.400005310181)) ;
#79105=CARTESIAN_POINT('Ctrl Pts',(130.842036869421,-75.7204074847575,-199.400005310181)) ;
#79106=CARTESIAN_POINT('Ctrl Pts',(130.789053275896,-75.7246379642313,-199.400005310181)) ;
#79107=CARTESIAN_POINT('Ctrl Pts',(130.736014303355,-75.7289657007846,-199.402812299913)) ;
#79108=CARTESIAN_POINT('Ctrl Pts',(130.488691675152,-75.7495845976627,-199.429160168525)) ;
#79109=CARTESIAN_POINT('Ctrl Pts',(130.300185846525,-75.7665718200039,-199.487696240402)) ;
#79110=CARTESIAN_POINT('Ctrl Pts',(129.955758181003,-75.800235894582,-199.674048679986)) ;
#79111=CARTESIAN_POINT('Ctrl Pts',(129.803265972982,-75.8157826860376,-199.800274398092)) ;
#79112=CARTESIAN_POINT('Ctrl Pts',(129.555874234132,-75.8481973565873,-200.103770906374)) ;
#79113=CARTESIAN_POINT('Ctrl Pts',(129.463190942205,-75.8651690514804,-200.277938023653)) ;
#79114=CARTESIAN_POINT('Ctrl Pts',(129.349584642592,-75.898856639705,-200.65279261781)) ;
#79115=CARTESIAN_POINT('Ctrl Pts',(129.330079232436,-75.9144540804814,-200.849965531322)) ;
#79116=CARTESIAN_POINT('Ctrl Pts',(129.368016288118,-75.9468319620272,-201.2397602553)) ;
#79117=CARTESIAN_POINT('Ctrl Pts',(129.424747760915,-75.963788329165,-201.428627134975)) ;
#79118=CARTESIAN_POINT('Ctrl Pts',(129.607910594488,-75.9974982023313,-201.774949571655)) ;
#79119=CARTESIAN_POINT('Ctrl Pts',(129.73296496394,-76.01314644887,-201.928861605832)) ;
#79120=CARTESIAN_POINT('Ctrl Pts',(130.034407896328,-76.045488585227,-202.179017955619)) ;
#79121=CARTESIAN_POINT('Ctrl Pts',(130.207584873293,-76.0624298680528,-202.273172111748)) ;
#79122=CARTESIAN_POINT('Ctrl Pts',(130.581547837697,-76.0961608319643,-202.390242512836)) ;
#79123=CARTESIAN_POINT('Ctrl Pts',(130.77888951949,-76.111859804738,-202.411515470159)) ;
#79124=CARTESIAN_POINT('Ctrl Pts',(131.169161293525,-76.1441672804533,-202.376858921408)) ;
#79125=CARTESIAN_POINT('Ctrl Pts',(131.35834777257,-76.1610937619284,-202.321802659239)) ;
#79126=CARTESIAN_POINT('Ctrl Pts',(131.706413790785,-76.1948446602018,-202.141608759678)) ;
#79127=CARTESIAN_POINT('Ctrl Pts',(131.861643938923,-76.2105940614007,-202.017643661455)) ;
#79128=CARTESIAN_POINT('Ctrl Pts',(132.114349873871,-76.2428679937785,-201.718111005681)) ;
#79129=CARTESIAN_POINT('Ctrl Pts',(132.20985468799,-76.2597799920395,-201.545860256861)) ;
#79130=CARTESIAN_POINT('Ctrl Pts',(132.330125403464,-76.2935497087167,-201.172737556653)) ;
#79131=CARTESIAN_POINT('Ctrl Pts',(132.353035129703,-76.3093490409428,-200.975240991203)) ;
#79132=CARTESIAN_POINT('Ctrl Pts',(132.321405445704,-76.3415905723374,-200.584541352067)) ;
#79133=CARTESIAN_POINT('Ctrl Pts',(132.267894073625,-76.3584884363231,-200.395073371258)) ;
#79134=CARTESIAN_POINT('Ctrl Pts',(132.090445274992,-76.3922758978451,-200.045412367649)) ;
#79135=CARTESIAN_POINT('Ctrl Pts',(131.96748662106,-76.4081244833936,-199.888966462595)) ;
#79136=CARTESIAN_POINT('Ctrl Pts',(131.669719158122,-76.4403347738487,-199.63392326637)) ;
#79137=CARTESIAN_POINT('Ctrl Pts',(131.498328538328,-76.4572188789652,-199.537185300362)) ;
#79138=CARTESIAN_POINT('Ctrl Pts',(131.161010070314,-76.4878437443242,-199.425563939749)) ;
#79139=CARTESIAN_POINT('Ctrl Pts',(131.001940017472,-76.5013900044752,-199.400005310181)) ;
#79140=CARTESIAN_POINT('Ctrl Pts',(130.842036869421,-76.5141574847575,-199.400005310181)) ;
#79141=CARTESIAN_POINT('Origin',(130.842036869422,-75.6433781549656,-200.900005310181)) ;
#79142=CARTESIAN_POINT('',(130.842036869422,-77.3079074847574,-199.400005310181)) ;
#79143=CARTESIAN_POINT('',(130.842036869422,-76.9050535907517,-199.400005310181)) ;
#79144=CARTESIAN_POINT('',(130.842036869422,-75.6433781549656,-199.400005310181)) ;
#79145=CARTESIAN_POINT('Ctrl Pts',(130.842036869422,-76.9050535907517,-199.400005310181)) ;
#79146=CARTESIAN_POINT('Ctrl Pts',(130.973277756236,-76.8945746511246,-199.400005310181)) ;
#79147=CARTESIAN_POINT('Ctrl Pts',(131.104164513265,-76.883554604073,-199.417221298495)) ;
#79148=CARTESIAN_POINT('Ctrl Pts',(131.42316821846,-76.8552478784647,-199.502966623318)) ;
#79149=CARTESIAN_POINT('Ctrl Pts',(131.602820838047,-76.8379560643228,-199.592085937357)) ;
#79150=CARTESIAN_POINT('Ctrl Pts',(131.912295362626,-76.8053273979256,-199.831515893817)) ;
#79151=CARTESIAN_POINT('Ctrl Pts',(132.040530630802,-76.7902332168997,-199.97765127425)) ;
#79152=CARTESIAN_POINT('Ctrl Pts',(132.237649557133,-76.756738893529,-200.315493307942)) ;
#79153=CARTESIAN_POINT('Ctrl Pts',(132.302667737018,-76.7394503735366,-200.505087687405)) ;
#79154=CARTESIAN_POINT('Ctrl Pts',(132.354348630853,-76.7067785325167,-200.892871149926)) ;
#79155=CARTESIAN_POINT('Ctrl Pts',(132.342762418159,-76.6917106911163,-201.086984832368)) ;
#79156=CARTESIAN_POINT('Ctrl Pts',(132.2458886052,-76.6584315923737,-201.463654223975)) ;
#79157=CARTESIAN_POINT('Ctrl Pts',(132.160197310018,-76.6413355443219,-201.642274951503)) ;
#79158=CARTESIAN_POINT('Ctrl Pts',(131.925793584997,-76.6085994180286,-201.955177264194)) ;
#79159=CARTESIAN_POINT('Ctrl Pts',(131.77984294802,-76.5934170441698,-202.086780793741)) ;
#79160=CARTESIAN_POINT('Ctrl Pts',(131.444367472244,-76.5599854470804,-202.28771649062)) ;
#79161=CARTESIAN_POINT('Ctrl Pts',(131.257750790847,-76.5428742303957,-202.354562487653)) ;
#79162=CARTESIAN_POINT('Ctrl Pts',(130.871128061817,-76.5100950834768,-202.412290164846)) ;
#79163=CARTESIAN_POINT('Ctrl Pts',(130.674983186419,-76.4949496843938,-202.403316448077)) ;
#79164=CARTESIAN_POINT('Ctrl Pts',(130.29516011843,-76.4615532102009,-202.310507293421)) ;
#79165=CARTESIAN_POINT('Ctrl Pts',(130.115325229674,-76.4444271428584,-202.22683957285)) ;
#79166=CARTESIAN_POINT('Ctrl Pts',(129.799803199283,-76.4116047496094,-201.99615201914)) ;
#79167=CARTESIAN_POINT('Ctrl Pts',(129.666695505079,-76.3964933948748,-201.852035070149)) ;
#79168=CARTESIAN_POINT('Ctrl Pts',(129.461705145776,-76.363133274824,-201.519134287027)) ;
#79169=CARTESIAN_POINT('Ctrl Pts',(129.392533140982,-76.3459927355846,-201.333113826507)) ;
#79170=CARTESIAN_POINT('Ctrl Pts',(129.330252747718,-76.3131269832385,-200.947292225973)) ;
#79171=CARTESIAN_POINT('Ctrl Pts',(129.336833153221,-76.2980465000572,-200.751383852506)) ;
#79172=CARTESIAN_POINT('Ctrl Pts',(129.424883567968,-76.264723917436,-200.370515086616)) ;
#79173=CARTESIAN_POINT('Ctrl Pts',(129.506446128229,-76.2475693434764,-200.189451187835)) ;
#79174=CARTESIAN_POINT('Ctrl Pts',(129.733285788991,-76.2146602341759,-199.871249254266)) ;
#79175=CARTESIAN_POINT('Ctrl Pts',(129.875521313557,-76.1996072313484,-199.736598692578)) ;
#79176=CARTESIAN_POINT('Ctrl Pts',(130.205750886396,-76.1663233112515,-199.527463459781)) ;
#79177=CARTESIAN_POINT('Ctrl Pts',(130.391129269758,-76.1491551949364,-199.455907517061)) ;
#79178=CARTESIAN_POINT('Ctrl Pts',(130.670105432118,-76.1252757574679,-199.407391615755)) ;
#79179=CARTESIAN_POINT('Ctrl Pts',(130.756081559722,-76.1181666996718,-199.400005310181)) ;
#79180=CARTESIAN_POINT('Ctrl Pts',(130.842036869422,-76.1113035907516,-199.400005310181)) ;
#79181=CARTESIAN_POINT('Ctrl Pts',(130.842036869421,-76.5141574847575,-199.400005310181)) ;
#79182=CARTESIAN_POINT('Ctrl Pts',(130.805260101874,-76.5170939288503,-199.400005310181)) ;
#79183=CARTESIAN_POINT('Ctrl Pts',(130.768446344966,-76.5200780567153,-199.401357787018)) ;
#79184=CARTESIAN_POINT('Ctrl Pts',(130.537271994658,-76.5391002762126,-199.418413557827)) ;
#79185=CARTESIAN_POINT('Ctrl Pts',(130.347557096745,-76.5559710200978,-199.470508809946)) ;
#79186=CARTESIAN_POINT('Ctrl Pts',(129.996444879957,-76.5897909265991,-199.645435083595)) ;
#79187=CARTESIAN_POINT('Ctrl Pts',(129.838884319023,-76.6057353618368,-199.767469352618)) ;
#79188=CARTESIAN_POINT('Ctrl Pts',(129.581710192247,-76.6378866870249,-200.063615659322)) ;
#79189=CARTESIAN_POINT('Ctrl Pts',(129.48385222616,-76.6547444854666,-200.234212888455)) ;
#79190=CARTESIAN_POINT('Ctrl Pts',(129.359505721472,-76.6881636884534,-200.601257419495)) ;
#79191=CARTESIAN_POINT('Ctrl Pts',(129.333434136973,-76.7038450753353,-200.793982602854)) ;
#79192=CARTESIAN_POINT('Ctrl Pts',(129.356031997873,-76.7358905682875,-201.18596811064)) ;
#79193=CARTESIAN_POINT('Ctrl Pts',(129.407341104038,-76.7531804135556,-201.381257572453)) ;
#79194=CARTESIAN_POINT('Ctrl Pts',(129.580292633447,-76.7870465825427,-201.733767158146)) ;
#79195=CARTESIAN_POINT('Ctrl Pts',(129.697743348234,-76.8027593414652,-201.888803616562)) ;
#79196=CARTESIAN_POINT('Ctrl Pts',(129.990270832118,-76.8347813779517,-202.150805152778)) ;
#79197=CARTESIAN_POINT('Ctrl Pts',(130.164427716409,-76.8520696019562,-202.253083793321)) ;
#79198=CARTESIAN_POINT('Ctrl Pts',(130.535734909097,-76.8859472142279,-202.380999886652)) ;
#79199=CARTESIAN_POINT('Ctrl Pts',(130.728367360873,-76.9016902851713,-202.408055647389)) ;
#79200=CARTESIAN_POINT('Ctrl Pts',(131.120596328859,-76.9336900193736,-202.387429123056)) ;
#79201=CARTESIAN_POINT('Ctrl Pts',(131.316234964971,-76.9509766065318,-202.337061511149)) ;
#79202=CARTESIAN_POINT('Ctrl Pts',(131.669706269178,-76.9848649572559,-202.165761083734)) ;
#79203=CARTESIAN_POINT('Ctrl Pts',(131.825339272788,-77.0006372432278,-202.049030903486)) ;
#79204=CARTESIAN_POINT('Ctrl Pts',(132.088820735292,-77.0326157990592,-201.757660987844)) ;
#79205=CARTESIAN_POINT('Ctrl Pts',(132.19196169619,-77.0499007470333,-201.58390231817)) ;
#79206=CARTESIAN_POINT('Ctrl Pts',(132.321624870104,-77.0837991688935,-201.21305816541)) ;
#79207=CARTESIAN_POINT('Ctrl Pts',(132.34956107743,-77.0995995474399,-201.020508531354)) ;
#79208=CARTESIAN_POINT('Ctrl Pts',(132.330697244536,-77.1315580160005,-200.628066253989)) ;
#79209=CARTESIAN_POINT('Ctrl Pts',(132.28117262879,-77.1488413339024,-200.432119382427)) ;
#79210=CARTESIAN_POINT('Ctrl Pts',(132.111349949548,-77.1827491959449,-200.077791610206)) ;
#79211=CARTESIAN_POINT('Ctrl Pts',(131.995263067737,-77.1985765294972,-199.921625849429)) ;
#79212=CARTESIAN_POINT('Ctrl Pts',(131.704929039509,-77.2305159670289,-199.656826323022)) ;
#79213=CARTESIAN_POINT('Ctrl Pts',(131.531529005047,-77.2477976737595,-199.552917543089)) ;
#79214=CARTESIAN_POINT('Ctrl Pts',(131.181874606249,-77.2798123464763,-199.429055232196)) ;
#79215=CARTESIAN_POINT('Ctrl Pts',(131.012501544664,-77.2942967184498,-199.400005310181)) ;
#79216=CARTESIAN_POINT('Ctrl Pts',(130.842036869422,-77.3079074847575,-199.400005310181)) ;
#79217=CARTESIAN_POINT('Origin',(130.842036869422,-75.6433781549656,-200.900005310181)) ;
#79218=CARTESIAN_POINT('',(130.842036869422,-78.1016574847575,-199.400005310181)) ;
#79219=CARTESIAN_POINT('',(130.842036869422,-77.6988035907517,-199.400005310181)) ;
#79220=CARTESIAN_POINT('',(130.842036869422,-75.6433781549656,-199.400005310181)) ;
#79221=CARTESIAN_POINT('',(130.148682626495,-78.162636333848,-199.569870018636)) ;
#79222=CARTESIAN_POINT('Ctrl Pts',(130.842036869422,-78.1016574847575,-199.400005310181)) ;
#79223=CARTESIAN_POINT('Ctrl Pts',(130.826012984664,-78.1029369131814,-199.400005310181)) ;
#79224=CARTESIAN_POINT('Ctrl Pts',(130.809980207002,-78.1042255435838,-199.40026207386)) ;
#79225=CARTESIAN_POINT('Ctrl Pts',(130.682617796906,-78.1145299262998,-199.404347603704)) ;
#79226=CARTESIAN_POINT('Ctrl Pts',(130.572056402493,-78.12388553057,-199.420306899202)) ;
#79227=CARTESIAN_POINT('Ctrl Pts',(130.354846362033,-78.1430979579179,-199.476826662743)) ;
#79228=CARTESIAN_POINT('Ctrl Pts',(130.248972434197,-78.1528997109598,-199.517592356254)) ;
#79229=CARTESIAN_POINT('Ctrl Pts',(130.148682626494,-78.1626363338481,-199.569870018636)) ;
#79230=CARTESIAN_POINT('',(131.596354821607,-78.162636333848,-202.196540858098)) ;
#79231=CARTESIAN_POINT('Origin',(130.842036869422,-78.162636333848,-200.900005310181)) ;
#79232=CARTESIAN_POINT('Ctrl Pts',(131.596354821608,-78.1626363338481,-202.196540858097)) ;
#79233=CARTESIAN_POINT('Ctrl Pts',(131.49689101871,-78.1527807895855,-202.254408405376)) ;
#79234=CARTESIAN_POINT('Ctrl Pts',(131.39110873996,-78.1428057769923,-202.300634073335)) ;
#79235=CARTESIAN_POINT('Ctrl Pts',(131.172260974558,-78.1231163253183,-202.367623431803)) ;
#79236=CARTESIAN_POINT('Ctrl Pts',(131.059986449382,-78.1134630724344,-202.388446632887)) ;
#79237=CARTESIAN_POINT('Ctrl Pts',(130.754280448219,-78.0883486428074,-202.409772490022)) ;
#79238=CARTESIAN_POINT('Ctrl Pts',(130.561333404588,-78.0728041866019,-202.38604789494)) ;
#79239=CARTESIAN_POINT('Ctrl Pts',(130.188312935722,-78.0390081124059,-202.264733419426)) ;
#79240=CARTESIAN_POINT('Ctrl Pts',(130.012689248877,-78.0217109294338,-202.165725068183)) ;
#79241=CARTESIAN_POINT('Ctrl Pts',(129.715826498257,-77.9895282788732,-201.90933342916)) ;
#79242=CARTESIAN_POINT('Ctrl Pts',(129.595660741605,-77.974019492826,-201.756542963972)) ;
#79243=CARTESIAN_POINT('Ctrl Pts',(129.416527173312,-77.9402399793395,-201.407679358008)) ;
#79244=CARTESIAN_POINT('Ctrl Pts',(129.361697254571,-77.9229416709976,-201.213742270841)) ;
#79245=CARTESIAN_POINT('Ctrl Pts',(129.331700777835,-77.8907281445107,-200.822716875643)) ;
#79246=CARTESIAN_POINT('Ctrl Pts',(129.35408257953,-77.8752555553349,-200.629642407692)) ;
#79247=CARTESIAN_POINT('Ctrl Pts',(129.472740133472,-77.8414935896882,-200.255948589964)) ;
#79248=CARTESIAN_POINT('Ctrl Pts',(129.570427250837,-77.8241943253707,-200.079751562834)) ;
#79249=CARTESIAN_POINT('Ctrl Pts',(129.824553178997,-77.7919486768708,-199.781161321941)) ;
#79250=CARTESIAN_POINT('Ctrl Pts',(129.976443198279,-77.7765126636698,-199.659905991275)) ;
#79251=CARTESIAN_POINT('Ctrl Pts',(130.323834208348,-77.7427692720935,-199.478309452035)) ;
#79252=CARTESIAN_POINT('Ctrl Pts',(130.517212622459,-77.7254692521619,-199.422079025222)) ;
#79253=CARTESIAN_POINT('Ctrl Pts',(130.757947644041,-77.7055761044962,-199.401771180552)) ;
#79254=CARTESIAN_POINT('Ctrl Pts',(130.800013424201,-77.7021589562638,-199.400005310181)) ;
#79255=CARTESIAN_POINT('Ctrl Pts',(130.842036869421,-77.6988035907517,-199.400005310181)) ;
#79256=CARTESIAN_POINT('Origin',(130.842036869422,-75.6433781549656,-200.900005310181)) ;
#79257=CARTESIAN_POINT('Ctrl Pts',(130.842036869421,-77.6988035907517,-199.400005310181)) ;
#79258=CARTESIAN_POINT('Ctrl Pts',(130.992008831122,-77.6868290668776,-199.400005310181)) ;
#79259=CARTESIAN_POINT('Ctrl Pts',(131.141323533336,-77.6741634905891,-199.422486888103)) ;
#79260=CARTESIAN_POINT('Ctrl Pts',(131.475469354102,-77.6440672695971,-199.525783489103)) ;
#79261=CARTESIAN_POINT('Ctrl Pts',(131.652283192623,-77.6267667275403,-199.622020126052)) ;
#79262=CARTESIAN_POINT('Ctrl Pts',(131.952754395999,-77.5944531510418,-199.873658895021)) ;
#79263=CARTESIAN_POINT('Ctrl Pts',(132.075201405575,-77.5790907454146,-200.024564717812)) ;
#79264=CARTESIAN_POINT('Ctrl Pts',(132.259479675576,-77.5453877295651,-200.370339242824)) ;
#79265=CARTESIAN_POINT('Ctrl Pts',(132.317233347614,-77.5280869339979,-200.56309642236)) ;
#79266=CARTESIAN_POINT('Ctrl Pts',(132.353408227123,-77.4957375987893,-200.95326354207)) ;
#79267=CARTESIAN_POINT('Ctrl Pts',(132.334104045199,-77.4804118388597,-201.146631517833)) ;
#79268=CARTESIAN_POINT('Ctrl Pts',(132.22152570243,-77.4467306937986,-201.521831209849)) ;
#79269=CARTESIAN_POINT('Ctrl Pts',(132.126871825135,-77.4294299502341,-201.699303172619)) ;
#79270=CARTESIAN_POINT('Ctrl Pts',(131.877947072605,-77.3970437056544,-202.001808671817)) ;
#79271=CARTESIAN_POINT('Ctrl Pts',(131.728110265776,-77.3817541999581,-202.125551001611)) ;
#79272=CARTESIAN_POINT('Ctrl Pts',(131.384099552374,-77.3480960890395,-202.312729734136)) ;
#79273=CARTESIAN_POINT('Ctrl Pts',(131.192029511511,-77.3307957413689,-202.372128762973)) ;
#79274=CARTESIAN_POINT('Ctrl Pts',(130.802370384407,-77.2983714823411,-202.411795458234)) ;
#79275=CARTESIAN_POINT('Ctrl Pts',(130.608835675341,-77.2831176049036,-202.394229680283)) ;
#79276=CARTESIAN_POINT('Ctrl Pts',(130.232808390015,-77.2494837181064,-202.285078235795)) ;
#79277=CARTESIAN_POINT('Ctrl Pts',(130.054640466163,-77.2321841497198,-202.192140090124)) ;
#79278=CARTESIAN_POINT('Ctrl Pts',(129.749950823865,-77.1997208259819,-201.94615774307)) ;
#79279=CARTESIAN_POINT('Ctrl Pts',(129.624809896354,-77.1845017022962,-201.79747424918)) ;
#79280=CARTESIAN_POINT('Ctrl Pts',(129.434516675332,-77.1508932519114,-201.455375560225)) ;
#79281=CARTESIAN_POINT('Ctrl Pts',(129.373353578203,-77.1335948863862,-201.26406104526)) ;
#79282=CARTESIAN_POINT('Ctrl Pts',(129.329930478591,-77.1010915117849,-200.874967008356)) ;
#79283=CARTESIAN_POINT('Ctrl Pts',(129.345626577679,-77.0859060069524,-200.68125218463)) ;
#79284=CARTESIAN_POINT('Ctrl Pts',(129.451098485901,-77.0523242226114,-200.304353329801)) ;
#79285=CARTESIAN_POINT('Ctrl Pts',(129.542190023052,-77.0350275239044,-200.125456456248)) ;
#79286=CARTESIAN_POINT('Ctrl Pts',(129.785004660559,-77.0024831856076,-199.818440058895)) ;
#79287=CARTESIAN_POINT('Ctrl Pts',(129.932452894176,-76.9873298951115,-199.691799819314)) ;
#79288=CARTESIAN_POINT('Ctrl Pts',(130.272493493307,-76.9537760181528,-199.498188024059)) ;
#79289=CARTESIAN_POINT('Ctrl Pts',(130.46298275716,-76.9364814902319,-199.435148629158)) ;
#79290=CARTESIAN_POINT('Ctrl Pts',(130.720672404424,-76.9148656030244,-199.403683739152)) ;
#79291=CARTESIAN_POINT('Ctrl Pts',(130.781382737284,-76.9098965250249,-199.400005310181)) ;
#79292=CARTESIAN_POINT('Ctrl Pts',(130.842036869422,-76.9050535907517,-199.400005310181)) ;
#79293=CARTESIAN_POINT('Ctrl Pts',(130.842036869422,-77.3079074847574,-199.400005310181)) ;
#79294=CARTESIAN_POINT('Ctrl Pts',(130.820046030699,-77.3096633451218,-199.400005310181)) ;
#79295=CARTESIAN_POINT('Ctrl Pts',(130.798039539999,-77.3114364490101,-199.400488901959)) ;
#79296=CARTESIAN_POINT('Ctrl Pts',(130.575996418083,-77.3294889515356,-199.410268832037)) ;
#79297=CARTESIAN_POINT('Ctrl Pts',(130.379778101036,-77.3467690742638,-199.459041510435)) ;
#79298=CARTESIAN_POINT('Ctrl Pts',(130.024690032456,-77.3806940629399,-199.62754651657)) ;
#79299=CARTESIAN_POINT('Ctrl Pts',(129.86805013415,-77.3965718782909,-199.743061024941)) ;
#79300=CARTESIAN_POINT('Ctrl Pts',(129.602080452281,-77.428476275587,-200.032471506143)) ;
#79301=CARTESIAN_POINT('Ctrl Pts',(129.497490180716,-77.4457548483642,-200.205550007105)) ;
#79302=CARTESIAN_POINT('Ctrl Pts',(129.364884363641,-77.4796875897104,-200.575605103068)) ;
#79303=CARTESIAN_POINT('Ctrl Pts',(129.335466147829,-77.4955889433358,-200.768015612496)) ;
#79304=CARTESIAN_POINT('Ctrl Pts',(129.351364949874,-77.5274772554681,-201.160807389023)) ;
#79305=CARTESIAN_POINT('Ctrl Pts',(129.399469184275,-77.5447543179783,-201.357264257698)) ;
#79306=CARTESIAN_POINT('Ctrl Pts',(129.566803157659,-77.5786943134002,-201.713025332201)) ;
#79307=CARTESIAN_POINT('Ctrl Pts',(129.681809956479,-77.5946180886615,-201.87008589028)) ;
#79308=CARTESIAN_POINT('Ctrl Pts',(129.970399781909,-77.6264912206868,-202.137091466825)) ;
#79309=CARTESIAN_POINT('Ctrl Pts',(130.143191170662,-77.6437668171255,-202.242284895348)) ;
#79310=CARTESIAN_POINT('Ctrl Pts',(130.512913843575,-77.6777135976496,-202.376117744342)) ;
#79311=CARTESIAN_POINT('Ctrl Pts',(130.705266466733,-77.6936586984264,-202.406153605062)) ;
#79312=CARTESIAN_POINT('Ctrl Pts',(131.098200371139,-77.7255175164878,-202.391489719301)) ;
#79313=CARTESIAN_POINT('Ctrl Pts',(131.294866508558,-77.7427916945635,-202.343977918736)) ;
#79314=CARTESIAN_POINT('Ctrl Pts',(131.651221821218,-77.7767448194291,-202.177681578418)) ;
#79315=CARTESIAN_POINT('Ctrl Pts',(131.808654563925,-77.7927101744347,-202.063123903972)) ;
#79316=CARTESIAN_POINT('Ctrl Pts',(132.07657487055,-77.8245555059074,-201.775261153286)) ;
#79317=CARTESIAN_POINT('Ctrl Pts',(132.182300787846,-77.8418283159611,-201.602725225993)) ;
#79318=CARTESIAN_POINT('Ctrl Pts',(132.317218105444,-77.8757873712274,-201.233298022712)) ;
#79319=CARTESIAN_POINT('Ctrl Pts',(132.347799699357,-77.8917719375526,-201.040996502765)) ;
#79320=CARTESIAN_POINT('Ctrl Pts',(132.334226538529,-77.9236045714227,-200.647938742724)) ;
#79321=CARTESIAN_POINT('Ctrl Pts',(132.287238405253,-77.9408760656535,-200.451089308365)) ;
#79322=CARTESIAN_POINT('Ctrl Pts',(132.121859081654,-77.9748406628289,-200.094210472838)) ;
#79323=CARTESIAN_POINT('Ctrl Pts',(132.007697746346,-77.9908434287853,-199.936449239791)) ;
#79324=CARTESIAN_POINT('Ctrl Pts',(131.720477474982,-78.0226641162253,-199.667722993288)) ;
#79325=CARTESIAN_POINT('Ctrl Pts',(131.548168129765,-78.0399343480179,-199.561528015344)) ;
#79326=CARTESIAN_POINT('Ctrl Pts',(131.194068406748,-78.0725178154868,-199.431199462941)) ;
#79327=CARTESIAN_POINT('Ctrl Pts',(131.018673974061,-78.0875538803064,-199.400005310181)) ;
#79328=CARTESIAN_POINT('Ctrl Pts',(130.842036869422,-78.1016574847574,-199.400005310181)) ;
#79329=CARTESIAN_POINT('Origin',(130.842036869422,-80.5295274127545,-200.900005310181)) ;
#79330=CARTESIAN_POINT('Ctrl Pts',(130.842036869422,-77.8506211627547,-202.652605310181)) ;
#79331=CARTESIAN_POINT('Ctrl Pts',(130.644451329195,-77.8371187371731,-202.652605310181)) ;
#79332=CARTESIAN_POINT('Ctrl Pts',(130.448097214639,-77.8227548518017,-202.619198734178)) ;
#79333=CARTESIAN_POINT('Ctrl Pts',(130.040901161784,-77.7908800902098,-202.476185390008)) ;
#79334=CARTESIAN_POINT('Ctrl Pts',(129.838174909486,-77.7736101243252,-202.355496502983)) ;
#79335=CARTESIAN_POINT('Ctrl Pts',(129.498362301134,-77.7416703239782,-202.047507444084)) ;
#79336=CARTESIAN_POINT('Ctrl Pts',(129.362281696203,-77.7259000849022,-201.865706510437)) ;
#79337=CARTESIAN_POINT('Ctrl Pts',(129.162621889232,-77.6920386786955,-201.452902951119)) ;
#79338=CARTESIAN_POINT('Ctrl Pts',(129.103964484698,-77.6747666285661,-201.224451918021)) ;
#79339=CARTESIAN_POINT('Ctrl Pts',(129.080106017582,-77.642799764517,-200.766552532796)) ;
#79340=CARTESIAN_POINT('Ctrl Pts',(129.111757813305,-77.6270671276914,-200.541712232754)) ;
#79341=CARTESIAN_POINT('Ctrl Pts',(129.261129496703,-77.5932194816432,-200.108280007658)) ;
#79342=CARTESIAN_POINT('Ctrl Pts',(129.380527623304,-77.5759453843576,-199.904958648707)) ;
#79343=CARTESIAN_POINT('Ctrl Pts',(129.686301058074,-77.5439500369427,-199.563415459841)) ;
#79344=CARTESIAN_POINT('Ctrl Pts',(129.867209754028,-77.528256224698,-199.426255935562)) ;
#79345=CARTESIAN_POINT('Ctrl Pts',(130.278573687824,-77.4944232819949,-199.224126123784)) ;
#79346=CARTESIAN_POINT('Ctrl Pts',(130.506500212819,-77.4771471983583,-199.164059948942)) ;
#79347=CARTESIAN_POINT('Ctrl Pts',(130.964032215596,-77.4451219218751,-199.137250947671)) ;
#79348=CARTESIAN_POINT('Ctrl Pts',(131.189012232965,-77.4294680618709,-199.167429429727)) ;
#79349=CARTESIAN_POINT('Ctrl Pts',(131.62320958988,-77.3956508170102,-199.313879908351)) ;
#79350=CARTESIAN_POINT('Ctrl Pts',(131.827186768078,-77.3783728346266,-199.431831999971)) ;
#79351=CARTESIAN_POINT('Ctrl Pts',(132.170655099965,-77.3463161635726,-199.735124169881)) ;
#79352=CARTESIAN_POINT('Ctrl Pts',(132.309018835436,-77.3307032671394,-199.915037539806)) ;
#79353=CARTESIAN_POINT('Ctrl Pts',(132.513895580475,-77.2969027664325,-200.324788921932)) ;
#79354=CARTESIAN_POINT('Ctrl Pts',(132.575527443354,-77.2796230028992,-200.552120766877)) ;
#79355=CARTESIAN_POINT('Ctrl Pts',(132.605622241063,-77.2475334590931,-201.009232193585)) ;
#79356=CARTESIAN_POINT('Ctrl Pts',(132.577083364891,-77.2319623982045,-201.234368161112)) ;
#79357=CARTESIAN_POINT('Ctrl Pts',(132.433881243309,-77.1981797398566,-201.669404915484)) ;
#79358=CARTESIAN_POINT('Ctrl Pts',(132.317540721715,-77.1808983460219,-201.874099548761)) ;
#79359=CARTESIAN_POINT('Ctrl Pts',(132.017012961559,-77.1487744466078,-202.219696711894)) ;
#79360=CARTESIAN_POINT('Ctrl Pts',(131.838203763758,-77.1332459297227,-202.359397169411)) ;
#79361=CARTESIAN_POINT('Ctrl Pts',(131.430249263693,-77.0994822634179,-202.567310685746)) ;
#79362=CARTESIAN_POINT('Ctrl Pts',(131.203588819781,-77.0821994266498,-202.630672025349)) ;
#79363=CARTESIAN_POINT('Ctrl Pts',(130.928130107247,-77.0627993718329,-202.651021002246)) ;
#79364=CARTESIAN_POINT('Ctrl Pts',(130.885062091297,-77.0598113822456,-202.652605310181)) ;
#79365=CARTESIAN_POINT('Ctrl Pts',(130.842036869423,-77.0568711627547,-202.652605310181)) ;
#79366=CARTESIAN_POINT('Ctrl Pts',(130.842036869423,-77.1560899127545,-202.652605310181)) ;
#79367=CARTESIAN_POINT('Ctrl Pts',(130.899863916809,-77.1600416462823,-202.652605310181)) ;
#79368=CARTESIAN_POINT('Ctrl Pts',(130.957751472884,-77.1640785216738,-202.649743499313)) ;
#79369=CARTESIAN_POINT('Ctrl Pts',(131.24683297456,-77.1846473603666,-202.620992047951)) ;
#79370=CARTESIAN_POINT('Ctrl Pts',(131.471277230816,-77.2019329520754,-202.552183031522)) ;
#79371=CARTESIAN_POINT('Ctrl Pts',(131.873460958087,-77.2355736049585,-202.334683455417)) ;
#79372=CARTESIAN_POINT('Ctrl Pts',(132.048757131248,-77.2508716670637,-202.19072395006)) ;
#79373=CARTESIAN_POINT('Ctrl Pts',(132.34040870828,-77.2832037156893,-201.838404233993)) ;
#79374=CARTESIAN_POINT('Ctrl Pts',(132.451572590196,-77.3004896097301,-201.631499513322)) ;
#79375=CARTESIAN_POINT('Ctrl Pts',(132.584388495721,-77.3341562011185,-201.1938590943)) ;
#79376=CARTESIAN_POINT('Ctrl Pts',(132.607674330953,-77.3494967795872,-200.968219965905)) ;
#79377=CARTESIAN_POINT('Ctrl Pts',(132.567039602767,-77.3817868708411,-200.512539643014)) ;
#79378=CARTESIAN_POINT('Ctrl Pts',(132.500409317965,-77.399072635403,-200.287190397148)) ;
#79379=CARTESIAN_POINT('Ctrl Pts',(132.28674768475,-77.4327637742788,-199.882678163347)) ;
#79380=CARTESIAN_POINT('Ctrl Pts',(132.144500759557,-77.4481474585741,-199.705970343403)) ;
#79381=CARTESIAN_POINT('Ctrl Pts',(131.794872857357,-77.4803969309762,-199.410737405653)) ;
#79382=CARTESIAN_POINT('Ctrl Pts',(131.588842742789,-77.4976821851599,-199.297484642701)) ;
#79383=CARTESIAN_POINT('Ctrl Pts',(131.15223619477,-77.5313965183911,-199.160486127959)) ;
#79384=CARTESIAN_POINT('Ctrl Pts',(130.926800560358,-77.5468236025095,-199.135082754097)) ;
#79385=CARTESIAN_POINT('Ctrl Pts',(130.470527967021,-77.5790338459698,-199.17146675209)) ;
#79386=CARTESIAN_POINT('Ctrl Pts',(130.244365397702,-77.5963182578483,-199.236085712784)) ;
#79387=CARTESIAN_POINT('Ctrl Pts',(129.83772801225,-77.6300544744548,-199.446209282137)) ;
#79388=CARTESIAN_POINT('Ctrl Pts',(129.659724973282,-77.645524979993,-199.5868862514)) ;
#79389=CARTESIAN_POINT('Ctrl Pts',(129.361223280434,-77.6776974239309,-199.934033007447)) ;
#79390=CARTESIAN_POINT('Ctrl Pts',(129.246064167252,-77.6949807081504,-200.139244658745)) ;
#79391=CARTESIAN_POINT('Ctrl Pts',(129.105238669955,-77.7287375427082,-200.57488795491)) ;
#79392=CARTESIAN_POINT('Ctrl Pts',(129.077900326764,-77.7442512433349,-200.800138432473)) ;
#79393=CARTESIAN_POINT('Ctrl Pts',(129.110402356064,-77.7763873453171,-201.256934052676)) ;
#79394=CARTESIAN_POINT('Ctrl Pts',(129.173179088576,-77.7936692603424,-201.4838231606)) ;
#79395=CARTESIAN_POINT('Ctrl Pts',(129.380065789546,-77.8274454955802,-201.892386906941)) ;
#79396=CARTESIAN_POINT('Ctrl Pts',(129.519313614305,-77.8430019422771,-202.071569910934)) ;
#79397=CARTESIAN_POINT('Ctrl Pts',(129.864190902294,-77.8751031773022,-202.37303491588)) ;
#79398=CARTESIAN_POINT('Ctrl Pts',(130.068643846436,-77.8923835224096,-202.48992187722)) ;
#79399=CARTESIAN_POINT('Ctrl Pts',(130.468250156428,-77.923445898564,-202.622558528809)) ;
#79400=CARTESIAN_POINT('Ctrl Pts',(130.654644951822,-77.9370340899242,-202.652605310181)) ;
#79401=CARTESIAN_POINT('Ctrl Pts',(130.842036869422,-77.9498399127545,-202.652605310181)) ;
#79402=CARTESIAN_POINT('Origin',(128.967036869422,-80.3871372990547,-194.819931163313)) ;
#79403=CARTESIAN_POINT('',(128.842036869421,-80.3871372990547,-205.37875531018)) ;
#79404=CARTESIAN_POINT('',(128.967036869421,-80.5121372990547,-205.37875531018)) ;
#79405=CARTESIAN_POINT('Origin',(128.967036869421,-80.3871372990547,-205.37875531018)) ;
#79406=CARTESIAN_POINT('',(128.967036869421,-80.5121372990547,-204.676255310181)) ;
#79407=CARTESIAN_POINT('',(128.967036869422,-80.5121372990547,-194.819931163313)) ;
#79408=CARTESIAN_POINT('',(128.842036869421,-80.3871372990547,-204.676255310181)) ;
#79409=CARTESIAN_POINT('Origin',(128.967036869421,-80.3871372990547,-204.676255310181)) ;
#79410=CARTESIAN_POINT('',(128.842036869422,-80.3871372990547,-194.819931163313)) ;
#79411=CARTESIAN_POINT('Origin',(131.540536869422,-80.5756372990547,-204.676255310181)) ;
#79412=CARTESIAN_POINT('',(131.540536869422,-80.5121372990547,-204.676255310181)) ;
#79413=CARTESIAN_POINT('',(131.477036869422,-80.5756372990547,-204.676255310181)) ;
#79414=CARTESIAN_POINT('Origin',(131.540536869422,-80.5756372990547,-204.676255310181)) ;
#79415=CARTESIAN_POINT('',(131.540536869422,-80.3871372990547,-204.551255310181)) ;
#79416=CARTESIAN_POINT('Origin',(131.540536869422,-80.3871372990547,-204.676255310181)) ;
#79417=CARTESIAN_POINT('',(131.352036869423,-80.5756372990547,-204.551255310181)) ;
#79418=CARTESIAN_POINT('Origin',(131.540536869422,-80.5756372990547,-204.551255310181)) ;
#79419=CARTESIAN_POINT('Origin',(131.352036869422,-80.5756372990547,-204.676255310181)) ;
#79420=CARTESIAN_POINT('Origin',(128.857661869421,-80.3871372990547,-204.676255310181)) ;
#79421=CARTESIAN_POINT('',(132.717036869422,-80.5121372990547,-204.676255310181)) ;
#79422=CARTESIAN_POINT('',(132.717036869422,-80.3871372990547,-204.551255310181)) ;
#79423=CARTESIAN_POINT('Origin',(132.717036869422,-80.3871372990547,-204.676255310181)) ;
#79424=CARTESIAN_POINT('',(128.857661869421,-80.3871372990547,-204.551255310181)) ;
#79425=CARTESIAN_POINT('',(128.857661869421,-80.5121372990547,-204.676255310181)) ;
#79426=CARTESIAN_POINT('Origin',(131.540536869422,-80.5756372990547,-205.378755310181)) ;
#79427=CARTESIAN_POINT('',(131.477036869422,-80.5756372990547,-205.378755310181)) ;
#79428=CARTESIAN_POINT('',(131.540536869422,-80.5121372990547,-205.378755310181)) ;
#79429=CARTESIAN_POINT('Origin',(131.540536869422,-80.5756372990547,-205.378755310181)) ;
#79430=CARTESIAN_POINT('',(131.352036869422,-80.5756372990547,-205.503755310181)) ;
#79431=CARTESIAN_POINT('Origin',(131.352036869422,-80.5756372990547,-205.378755310181)) ;
#79432=CARTESIAN_POINT('',(131.540536869422,-80.3871372990547,-205.503755310181)) ;
#79433=CARTESIAN_POINT('Origin',(131.540536869422,-80.5756372990547,-205.503755310181)) ;
#79434=CARTESIAN_POINT('Origin',(131.540536869422,-80.3871372990547,-205.378755310181)) ;
#79435=CARTESIAN_POINT('Origin',(130.143536869423,-80.5756372990547,-204.676255310181)) ;
#79436=CARTESIAN_POINT('',(130.207036869423,-80.5756372990547,-204.676255310181)) ;
#79437=CARTESIAN_POINT('',(130.143536869423,-80.5121372990547,-204.676255310181)) ;
#79438=CARTESIAN_POINT('Origin',(130.143536869423,-80.5756372990547,-204.676255310181)) ;
#79439=CARTESIAN_POINT('',(130.332036869423,-80.5756372990547,-204.551255310181)) ;
#79440=CARTESIAN_POINT('Origin',(130.332036869423,-80.5756372990547,-204.676255310181)) ;
#79441=CARTESIAN_POINT('',(130.143536869423,-80.3871372990547,-204.551255310181)) ;
#79442=CARTESIAN_POINT('Origin',(130.143536869423,-80.5756372990547,-204.551255310181)) ;
#79443=CARTESIAN_POINT('Origin',(130.143536869423,-80.3871372990547,-204.676255310181)) ;
#79444=CARTESIAN_POINT('Origin',(130.332036869423,-78.8018322834461,-204.676255310181)) ;
#79445=CARTESIAN_POINT('',(130.207036869423,-84.5845282330442,-204.676255310181)) ;
#79446=CARTESIAN_POINT('',(130.332036869423,-84.5845282330442,-204.551255310181)) ;
#79447=CARTESIAN_POINT('Origin',(130.332036869423,-84.5845282330442,-204.676255310181)) ;
#79448=CARTESIAN_POINT('',(130.332036869423,-78.8018322834461,-204.551255310181)) ;
#79449=CARTESIAN_POINT('',(130.207036869423,-78.8018322834461,-204.676255310181)) ;
#79450=CARTESIAN_POINT('Origin',(130.842036869423,-84.5845282330442,-204.676255310181)) ;
#79451=CARTESIAN_POINT('',(131.477036869423,-84.5845282330442,-204.676255310181)) ;
#79452=CARTESIAN_POINT('',(131.352036869423,-84.5845282330442,-204.551255310181)) ;
#79453=CARTESIAN_POINT('Origin',(131.352036869423,-84.5845282330442,-204.676255310181)) ;
#79454=CARTESIAN_POINT('Origin',(130.842036869423,-84.5845282330442,-204.551255310181)) ;
#79455=CARTESIAN_POINT('Origin',(130.842036869423,-84.5845282330442,-204.676255310181)) ;
#79456=CARTESIAN_POINT('Origin',(131.352036869422,-81.0243322834461,-204.676255310181)) ;
#79457=CARTESIAN_POINT('',(131.352036869423,-81.0243322834461,-204.551255310181)) ;
#79458=CARTESIAN_POINT('',(131.477036869422,-81.0243322834461,-204.676255310181)) ;
#79459=CARTESIAN_POINT('Origin',(128.857661869421,-80.3871372990547,-204.676255310181)) ;
#79460=CARTESIAN_POINT('',(128.967036869421,-80.3871372990547,-204.551255310181)) ;
#79461=CARTESIAN_POINT('Origin',(128.967036869421,-80.3871372990547,-204.676255310181)) ;
#79462=CARTESIAN_POINT('',(128.857661869421,-80.5121372990547,-204.676255310181)) ;
#79463=CARTESIAN_POINT('',(128.857661869421,-80.3871372990547,-204.551255310181)) ;
#79464=CARTESIAN_POINT('Origin',(130.143536869422,-80.5756372990547,-205.37875531018)) ;
#79465=CARTESIAN_POINT('',(130.143536869422,-80.5121372990547,-205.37875531018)) ;
#79466=CARTESIAN_POINT('',(130.207036869422,-80.5756372990547,-205.37875531018)) ;
#79467=CARTESIAN_POINT('Origin',(130.143536869422,-80.5756372990547,-205.37875531018)) ;
#79468=CARTESIAN_POINT('',(130.143536869422,-80.3871372990547,-205.50375531018)) ;
#79469=CARTESIAN_POINT('Origin',(130.143536869422,-80.3871372990547,-205.37875531018)) ;
#79470=CARTESIAN_POINT('',(130.332036869422,-80.5756372990547,-205.50375531018)) ;
#79471=CARTESIAN_POINT('Origin',(130.143536869422,-80.5756372990547,-205.50375531018)) ;
#79472=CARTESIAN_POINT('Origin',(130.332036869422,-80.5756372990547,-205.37875531018)) ;
#79473=CARTESIAN_POINT('Origin',(128.857661869421,-80.3871372990547,-205.37875531018)) ;
#79474=CARTESIAN_POINT('',(128.967036869421,-80.3871372990547,-205.50375531018)) ;
#79475=CARTESIAN_POINT('Origin',(128.967036869421,-80.3871372990547,-205.37875531018)) ;
#79476=CARTESIAN_POINT('',(128.857661869421,-80.3871372990547,-205.50375531018)) ;
#79477=CARTESIAN_POINT('',(128.857661869421,-80.5121372990547,-205.37875531018)) ;
#79478=CARTESIAN_POINT('Origin',(131.352036869422,-85.691582283446,-205.378755310181)) ;
#79479=CARTESIAN_POINT('',(131.477036869422,-84.5845282330442,-205.378755310181)) ;
#79480=CARTESIAN_POINT('',(131.352036869422,-84.5845282330442,-205.503755310181)) ;
#79481=CARTESIAN_POINT('Origin',(131.352036869422,-84.5845282330442,-205.378755310181)) ;
#79482=CARTESIAN_POINT('',(131.352036869422,-85.691582283446,-205.503755310181)) ;
#79483=CARTESIAN_POINT('',(131.477036869422,-85.691582283446,-205.378755310181)) ;
#79484=CARTESIAN_POINT('Origin',(130.842036869423,-84.5845282330442,-205.37875531018)) ;
#79485=CARTESIAN_POINT('',(130.207036869422,-84.5845282330442,-205.37875531018)) ;
#79486=CARTESIAN_POINT('',(130.332036869423,-84.5845282330442,-205.50375531018)) ;
#79487=CARTESIAN_POINT('Origin',(130.332036869423,-84.5845282330442,-205.37875531018)) ;
#79488=CARTESIAN_POINT('Origin',(130.842036869423,-84.5845282330442,-205.50375531018)) ;
#79489=CARTESIAN_POINT('Origin',(130.842036869423,-84.5845282330442,-205.37875531018)) ;
#79490=CARTESIAN_POINT('Origin',(130.332036869422,-83.469082283446,-205.37875531018)) ;
#79491=CARTESIAN_POINT('',(130.332036869422,-83.469082283446,-205.50375531018)) ;
#79492=CARTESIAN_POINT('',(130.207036869422,-83.469082283446,-205.37875531018)) ;
#79493=CARTESIAN_POINT('Origin',(130.143536869425,-80.5756372990547,-187.914255310181)) ;
#79494=CARTESIAN_POINT('',(130.207036869425,-80.5756372990547,-187.914255310181)) ;
#79495=CARTESIAN_POINT('',(130.143536869425,-80.5121372990547,-187.914255310181)) ;
#79496=CARTESIAN_POINT('Origin',(128.857661869421,-80.3871372990547,-205.37875531018)) ;
#79497=CARTESIAN_POINT('',(132.717036869421,-80.3871372990547,-205.503755310181)) ;
#79498=CARTESIAN_POINT('',(132.717036869421,-80.5121372990547,-205.378755310181)) ;
#79499=CARTESIAN_POINT('Origin',(132.717036869421,-80.3871372990547,-205.378755310181)) ;
#79500=CARTESIAN_POINT('',(128.857661869421,-80.5121372990547,-205.37875531018)) ;
#79501=CARTESIAN_POINT('',(128.857661869421,-80.3871372990547,-205.50375531018)) ;
#79502=CARTESIAN_POINT('Origin',(131.540536869425,-80.5756372990547,-188.739755310182)) ;
#79503=CARTESIAN_POINT('',(131.477036869425,-80.5756372990547,-188.739755310182)) ;
#79504=CARTESIAN_POINT('',(131.540536869425,-80.5121372990547,-188.739755310182)) ;
#79505=CARTESIAN_POINT('Origin',(128.967036869421,-80.3871372990547,-205.37875531018)) ;
#79506=CARTESIAN_POINT('Origin',(128.967036869421,-80.3871372990547,-205.37875531018)) ;
#79507=CARTESIAN_POINT('Origin',(128.967036869421,-80.3871372990547,-204.676255310181)) ;
#79508=CARTESIAN_POINT('Origin',(128.967036869421,-80.3871372990547,-204.676255310181)) ;
#79509=CARTESIAN_POINT('Origin',(132.717036869422,-80.3871372990547,-199.185505310181)) ;
#79510=CARTESIAN_POINT('',(132.842036869421,-80.3871372990547,-205.378755310181)) ;
#79511=CARTESIAN_POINT('Origin',(132.717036869421,-80.3871372990547,-205.378755310181)) ;
#79512=CARTESIAN_POINT('',(132.842036869422,-80.3871372990547,-204.676255310181)) ;
#79513=CARTESIAN_POINT('',(132.842036869422,-80.3871372990547,-199.185505310181)) ;
#79514=CARTESIAN_POINT('Origin',(132.717036869422,-80.3871372990547,-204.676255310181)) ;
#79515=CARTESIAN_POINT('',(132.717036869422,-80.5121372990547,-199.185505310181)) ;
#79516=CARTESIAN_POINT('Origin',(132.717036869421,-80.3871372990547,-205.378755310181)) ;
#79517=CARTESIAN_POINT('Origin',(132.717036869421,-80.3871372990547,-205.378755310181)) ;
#79518=CARTESIAN_POINT('Origin',(132.717036869422,-80.3871372990547,-204.676255310181)) ;
#79519=CARTESIAN_POINT('Origin',(132.717036869422,-80.3871372990547,-204.676255310181)) ;
#79520=CARTESIAN_POINT('Origin',(130.207036869425,-82.6795282330441,-187.088755310182)) ;
#79521=CARTESIAN_POINT('',(130.207036869422,-84.5845282330442,-205.503755310182)) ;
#79522=CARTESIAN_POINT('Origin',(128.967036869421,-77.019821262485,-204.676255310181)) ;
#79523=CARTESIAN_POINT('',(128.967036869421,-76.2556363338479,-204.551255310181)) ;
#79524=CARTESIAN_POINT('',(128.967036869421,-77.019821262485,-204.551255310181)) ;
#79525=CARTESIAN_POINT('',(128.842036869421,-76.2556363338479,-204.676255310181)) ;
#79526=CARTESIAN_POINT('Origin',(128.967036869421,-76.2556363338479,-204.676255310181)) ;
#79527=CARTESIAN_POINT('',(128.842036869421,-77.019821262485,-204.676255310181)) ;
#79528=CARTESIAN_POINT('Origin',(126.238286869421,-74.924136333848,-204.55125531018)) ;
#79529=CARTESIAN_POINT('',(132.717036869422,-76.2556363338479,-204.551255310181)) ;
#79530=CARTESIAN_POINT('',(132.717036869422,-75.051136333848,-204.551255310181)) ;
#79531=CARTESIAN_POINT('',(132.651420178853,-76.194136333848,-204.551255310181)) ;
#79532=CARTESIAN_POINT('Ctrl Pts',(132.717036869422,-76.2556363338479,-204.551255310181)) ;
#79533=CARTESIAN_POINT('Ctrl Pts',(132.697172914594,-76.2357723790203,-204.551255310181)) ;
#79534=CARTESIAN_POINT('Ctrl Pts',(132.675045468123,-76.2135667892559,-204.551255310181)) ;
#79535=CARTESIAN_POINT('Ctrl Pts',(132.651420178853,-76.194136333848,-204.551255310181)) ;
#79536=CARTESIAN_POINT('',(129.03265355999,-76.194136333848,-204.551255310181)) ;
#79537=CARTESIAN_POINT('',(126.492286869421,-76.194136333848,-204.55125531018)) ;
#79538=CARTESIAN_POINT('Ctrl Pts',(129.03265355999,-76.1941363338481,-204.551255310181)) ;
#79539=CARTESIAN_POINT('Ctrl Pts',(129.009028270719,-76.2135667892559,-204.551255310181)) ;
#79540=CARTESIAN_POINT('Ctrl Pts',(128.986900824248,-76.2357723790203,-204.551255310181)) ;
#79541=CARTESIAN_POINT('Ctrl Pts',(128.967036869421,-76.2556363338479,-204.551255310181)) ;
#79542=CARTESIAN_POINT('Origin',(132.717036869422,-75.051136333848,-204.676255310181)) ;
#79543=CARTESIAN_POINT('',(132.842036869422,-76.2556363338479,-204.676255310181)) ;
#79544=CARTESIAN_POINT('',(132.842036869422,-75.051136333848,-204.676255310181)) ;
#79545=CARTESIAN_POINT('Origin',(132.717036869422,-76.2556363338479,-204.676255310181)) ;
#79546=CARTESIAN_POINT('Origin',(132.842036869421,-75.178136333848,-209.631255310181)) ;
#79547=CARTESIAN_POINT('',(132.842036869421,-76.2556363338479,-205.378755310181)) ;
#79548=CARTESIAN_POINT('',(132.842036869421,-79.7183863338479,-205.378755310181)) ;
#79549=CARTESIAN_POINT('',(132.842036869421,-76.2556363338479,-205.265630310181)) ;
#79550=CARTESIAN_POINT('Origin',(131.477036869424,-80.5121372990547,-188.739755310181)) ;
#79551=CARTESIAN_POINT('Origin',(131.477036869424,-80.5121372990547,-188.739755310181)) ;
#79552=CARTESIAN_POINT('Origin',(131.477036869425,-87.1245282330441,-188.739755310182)) ;
#79553=CARTESIAN_POINT('',(131.477036869422,-84.5845282330442,-205.503755310182)) ;
#79554=CARTESIAN_POINT('Origin',(130.842036869423,-84.5845282330442,-200.106255310182)) ;
#79555=CARTESIAN_POINT('Origin',(132.717036869421,-79.7183863338479,-205.378755310181)) ;
#79556=CARTESIAN_POINT('',(132.717036869421,-76.2556363338479,-205.503755310181)) ;
#79557=CARTESIAN_POINT('',(132.717036869421,-79.7183863338479,-205.503755310181)) ;
#79558=CARTESIAN_POINT('Origin',(132.717036869421,-76.2556363338479,-205.378755310181)) ;
#79559=CARTESIAN_POINT('Origin',(128.967036869421,-81.687071262485,-205.37875531018)) ;
#79560=CARTESIAN_POINT('',(128.842036869421,-76.2556363338479,-205.37875531018)) ;
#79561=CARTESIAN_POINT('',(128.842036869421,-81.687071262485,-205.37875531018)) ;
#79562=CARTESIAN_POINT('',(128.967036869421,-76.2556363338479,-205.50375531018)) ;
#79563=CARTESIAN_POINT('Origin',(128.967036869421,-76.2556363338479,-205.37875531018)) ;
#79564=CARTESIAN_POINT('',(128.967036869421,-81.687071262485,-205.50375531018)) ;
#79565=CARTESIAN_POINT('Origin',(126.238286869421,-84.2586363338479,-205.50375531018)) ;
#79566=CARTESIAN_POINT('',(128.717036869421,-76.0056363338479,-205.50375531018)) ;
#79567=CARTESIAN_POINT('Origin',(128.717036869421,-76.2556363338479,-205.50375531018)) ;
#79568=CARTESIAN_POINT('',(126.96703686942,-76.0056363338479,-205.50375531018)) ;
#79569=CARTESIAN_POINT('',(126.238286869421,-76.0056363338479,-205.50375531018)) ;
#79570=CARTESIAN_POINT('',(126.96703686942,-75.8766363338479,-205.50375531018)) ;
#79571=CARTESIAN_POINT('',(126.96703686942,-81.6870712624849,-205.50375531018)) ;
#79572=CARTESIAN_POINT('',(134.717036869421,-75.8766363338479,-205.503755310181)) ;
#79573=CARTESIAN_POINT('',(126.492286869421,-75.8766363338479,-205.50375531018)) ;
#79574=CARTESIAN_POINT('',(134.717036869421,-76.0056363338479,-205.503755310181)) ;
#79575=CARTESIAN_POINT('',(134.717036869421,-79.7183863338479,-205.503755310181)) ;
#79576=CARTESIAN_POINT('',(132.967036869421,-76.0056363338479,-205.503755310181)) ;
#79577=CARTESIAN_POINT('',(126.238286869421,-76.0056363338479,-205.50375531018)) ;
#79578=CARTESIAN_POINT('Origin',(132.967036869421,-76.2556363338479,-205.503755310181)) ;
#79579=CARTESIAN_POINT('Origin',(128.842036869421,-79.1155061911221,-200.900107016445)) ;
#79580=CARTESIAN_POINT('',(128.842036869421,-76.2556363338479,-200.900056163313)) ;
#79581=CARTESIAN_POINT('Origin',(126.238286869423,-84.2586363338479,-197.24875531018)) ;
#79582=CARTESIAN_POINT('',(128.967036869422,-80.3871363338479,-197.248755310181)) ;
#79583=CARTESIAN_POINT('',(132.717036869423,-80.3871363338479,-197.248755310181)) ;
#79584=CARTESIAN_POINT('',(128.857661869423,-80.3871363338479,-197.248755310181)) ;
#79585=CARTESIAN_POINT('',(128.967036869422,-76.2556363338479,-197.248755310181)) ;
#79586=CARTESIAN_POINT('',(128.967036869422,-81.687071262485,-197.248755310181)) ;
#79587=CARTESIAN_POINT('',(129.032653559991,-76.194136333848,-197.248755310181)) ;
#79588=CARTESIAN_POINT('Ctrl Pts',(128.967036869422,-76.2556363338479,-197.248755310181)) ;
#79589=CARTESIAN_POINT('Ctrl Pts',(128.98690082425,-76.2357723790203,-197.248755310181)) ;
#79590=CARTESIAN_POINT('Ctrl Pts',(129.00902827072,-76.2135667892558,-197.248755310181)) ;
#79591=CARTESIAN_POINT('Ctrl Pts',(129.032653559991,-76.1941363338479,-197.248755310181)) ;
#79592=CARTESIAN_POINT('',(132.651420178854,-76.194136333848,-197.248755310181)) ;
#79593=CARTESIAN_POINT('',(126.492286869423,-76.194136333848,-197.24875531018)) ;
#79594=CARTESIAN_POINT('',(132.717036869423,-76.2556363338479,-197.248755310181)) ;
#79595=CARTESIAN_POINT('Ctrl Pts',(132.651420178854,-76.194136333848,-197.248755310181)) ;
#79596=CARTESIAN_POINT('Ctrl Pts',(132.675045468124,-76.2135667892558,-197.248755310181)) ;
#79597=CARTESIAN_POINT('Ctrl Pts',(132.697172914595,-76.2357723790203,-197.248755310181)) ;
#79598=CARTESIAN_POINT('Ctrl Pts',(132.717036869423,-76.2556363338479,-197.248755310181)) ;
#79599=CARTESIAN_POINT('',(132.717036869423,-79.7183863338479,-197.248755310181)) ;
#79600=CARTESIAN_POINT('Origin',(131.477036869424,-80.5121363338479,-188.739755310181)) ;
#79601=CARTESIAN_POINT('',(132.717036869423,-80.5121363338479,-197.123755310181)) ;
#79602=CARTESIAN_POINT('',(128.967036869422,-80.512136333848,-197.123755310181)) ;
#79603=CARTESIAN_POINT('',(128.857661869423,-80.512136333848,-197.123755310181)) ;
#79604=CARTESIAN_POINT('',(132.717036869423,-80.5121363338479,-196.421255310181)) ;
#79605=CARTESIAN_POINT('',(132.717036869422,-80.512136333848,-199.185505310181)) ;
#79606=CARTESIAN_POINT('',(128.967036869422,-80.512136333848,-196.42125531018)) ;
#79607=CARTESIAN_POINT('',(128.857661869422,-80.512136333848,-196.42125531018)) ;
#79608=CARTESIAN_POINT('',(128.967036869422,-80.512136333848,-194.819931163313)) ;
#79609=CARTESIAN_POINT('Origin',(126.238286869422,-74.6066363338479,-196.29625531018)) ;
#79610=CARTESIAN_POINT('',(132.717036869423,-80.3871363338479,-196.296255310181)) ;
#79611=CARTESIAN_POINT('',(128.967036869422,-80.3871363338479,-196.29625531018)) ;
#79612=CARTESIAN_POINT('',(128.857661869422,-80.3871363338479,-196.29625531018)) ;
#79613=CARTESIAN_POINT('',(132.717036869423,-76.2556363338479,-196.296255310181)) ;
#79614=CARTESIAN_POINT('',(132.717036869423,-74.8923863338479,-196.296255310181)) ;
#79615=CARTESIAN_POINT('',(132.967036869423,-76.0056363338479,-196.296255310181)) ;
#79616=CARTESIAN_POINT('Origin',(132.967036869423,-76.2556363338479,-196.296255310181)) ;
#79617=CARTESIAN_POINT('',(134.717036869422,-76.0056363338479,-196.296255310181)) ;
#79618=CARTESIAN_POINT('',(126.238286869422,-76.0056363338479,-196.29625531018)) ;
#79619=CARTESIAN_POINT('',(134.717036869422,-75.8766363338479,-196.296255310181)) ;
#79620=CARTESIAN_POINT('',(134.717036869422,-74.8923863338479,-196.296255310181)) ;
#79621=CARTESIAN_POINT('',(126.967036869422,-75.8766363338479,-196.29625531018)) ;
#79622=CARTESIAN_POINT('',(126.492286869422,-75.8766363338479,-196.29625531018)) ;
#79623=CARTESIAN_POINT('',(126.967036869422,-76.0056363338479,-196.29625531018)) ;
#79624=CARTESIAN_POINT('',(126.967036869422,-76.8610712624849,-196.29625531018)) ;
#79625=CARTESIAN_POINT('',(128.717036869422,-76.0056363338479,-196.29625531018)) ;
#79626=CARTESIAN_POINT('',(126.238286869422,-76.0056363338479,-196.29625531018)) ;
#79627=CARTESIAN_POINT('',(128.967036869422,-76.2556363338479,-196.29625531018)) ;
#79628=CARTESIAN_POINT('Origin',(128.717036869422,-76.2556363338479,-196.29625531018)) ;
#79629=CARTESIAN_POINT('',(128.967036869422,-76.861071262485,-196.29625531018)) ;
#79630=CARTESIAN_POINT('Origin',(126.238286869422,-75.1781363338479,-200.90000531018)) ;
#79631=CARTESIAN_POINT('',(126.967036869421,-75.1781363338479,-196.99475531018)) ;
#79632=CARTESIAN_POINT('',(126.96703686942,-75.1781363338479,-204.80525531018)) ;
#79633=CARTESIAN_POINT('',(126.967036869421,-75.1781363338479,-200.900056163312)) ;
#79634=CARTESIAN_POINT('',(134.717036869422,-75.1781363338479,-196.994755310181)) ;
#79635=CARTESIAN_POINT('',(126.492286869422,-75.1781363338479,-196.99475531018)) ;
#79636=CARTESIAN_POINT('',(134.717036869421,-75.1781363338479,-204.805255310181)) ;
#79637=CARTESIAN_POINT('',(134.717036869421,-75.1781363338479,-205.265630310181)) ;
#79638=CARTESIAN_POINT('',(126.492286869421,-75.1781363338479,-204.80525531018)) ;
#79639=CARTESIAN_POINT('Ctrl Pts',(129.538783258279,-75.1781363338479,-199.728196117098)) ;
#79640=CARTESIAN_POINT('Ctrl Pts',(129.45800656813,-75.1781363338479,-199.843248165079)) ;
#79641=CARTESIAN_POINT('Ctrl Pts',(129.392083038491,-75.1781363338479,-199.968013747906)) ;
#79642=CARTESIAN_POINT('Ctrl Pts',(129.295765628632,-75.1781363338479,-200.224210513459)) ;
#79643=CARTESIAN_POINT('Ctrl Pts',(129.264039116857,-75.1781363336273,-200.353975535856)) ;
#79644=CARTESIAN_POINT('Ctrl Pts',(129.237141221678,-75.1781363336273,-200.577407440569)) ;
#79645=CARTESIAN_POINT('Ctrl Pts',(129.233742341553,-75.1781363339454,-200.669408192917)) ;
#79646=CARTESIAN_POINT('Ctrl Pts',(129.246388555036,-75.1781363339454,-200.944817520171)) ;
#79647=CARTESIAN_POINT('Ctrl Pts',(129.28319680131,-75.1781363338479,-201.083489158714)) ;
#79648=CARTESIAN_POINT('Ctrl Pts',(129.349105122886,-75.1781363338479,-201.28766056179)) ;
#79649=CARTESIAN_POINT('Ctrl Pts',(129.403482219833,-75.1781363338479,-201.403236625849)) ;
#79650=CARTESIAN_POINT('Ctrl Pts',(129.471900051694,-75.1781363338479,-201.5105174728)) ;
#79651=CARTESIAN_POINT('Ctrl Pts',(132.182528457453,-75.1781363338479,-200.226891425003)) ;
#79652=CARTESIAN_POINT('Ctrl Pts',(132.131574767273,-75.1781363338479,-200.071657123996)) ;
#79653=CARTESIAN_POINT('Ctrl Pts',(132.055096968141,-75.1781363338479,-199.926049956735)) ;
#79654=CARTESIAN_POINT('Ctrl Pts',(131.886671256346,-75.1781363338479,-199.704076104489)) ;
#79655=CARTESIAN_POINT('Ctrl Pts',(131.769830068204,-75.1781363338479,-199.569294695449)) ;
#79656=CARTESIAN_POINT('Ctrl Pts',(131.470525930309,-75.1781363338479,-199.36014270823)) ;
#79657=CARTESIAN_POINT('Ctrl Pts',(131.341077459766,-75.1781363338479,-199.293181639218)) ;
#79658=CARTESIAN_POINT('Ctrl Pts',(131.057089712392,-75.1781363338479,-199.191077475863)) ;
#79659=CARTESIAN_POINT('Ctrl Pts',(130.90605206945,-75.1781363338479,-199.160428444176)) ;
#79660=CARTESIAN_POINT('Ctrl Pts',(130.749091630179,-75.1781363338479,-199.14987161743)) ;
#79661=CARTESIAN_POINT('Origin',(126.238286869422,-75.8766363338479,-196.99475531018)) ;
#79662=CARTESIAN_POINT('Origin',(126.967036869421,-75.8766363338479,-196.99475531018)) ;
#79663=CARTESIAN_POINT('Origin',(134.717036869422,-75.8766363338479,-196.994755310181)) ;
#79664=CARTESIAN_POINT('Origin',(126.238286869421,-75.8766363338479,-204.80525531018)) ;
#79665=CARTESIAN_POINT('Origin',(126.96703686942,-75.8766363338479,-204.80525531018)) ;
#79666=CARTESIAN_POINT('Origin',(134.717036869421,-75.8766363338479,-204.805255310181)) ;
#79667=CARTESIAN_POINT('Origin',(126.238286869423,-76.194136333848,-197.31225531018)) ;
#79668=CARTESIAN_POINT('',(132.552818265117,-76.1306363338479,-197.312255310181)) ;
#79669=CARTESIAN_POINT('Ctrl Pts',(132.552818265118,-76.1306363338479,-197.312255310181)) ;
#79670=CARTESIAN_POINT('Ctrl Pts',(132.553235902517,-76.1306363338479,-197.311832627558)) ;
#79671=CARTESIAN_POINT('Ctrl Pts',(132.553653540005,-76.1306405541772,-197.311409957672)) ;
#79672=CARTESIAN_POINT('Ctrl Pts',(132.561306890963,-76.1307952165411,-197.303665859274)) ;
#79673=CARTESIAN_POINT('Ctrl Pts',(132.568504138283,-76.1322072351016,-197.296404775943)) ;
#79674=CARTESIAN_POINT('Ctrl Pts',(132.582932569029,-76.137491469148,-197.282617198858)) ;
#79675=CARTESIAN_POINT('Ctrl Pts',(132.590067314198,-76.141343967398,-197.276182188304)) ;
#79676=CARTESIAN_POINT('Ctrl Pts',(132.60894050488,-76.1543405140709,-197.261267814067)) ;
#79677=CARTESIAN_POINT('Ctrl Pts',(132.619689006199,-76.1646337439611,-197.254884983358)) ;
#79678=CARTESIAN_POINT('Ctrl Pts',(132.637807265837,-76.1820606916733,-197.24953905352)) ;
#79679=CARTESIAN_POINT('Ctrl Pts',(132.644422115438,-76.1883808250967,-197.248755310181)) ;
#79680=CARTESIAN_POINT('Ctrl Pts',(132.651420178854,-76.194136333848,-197.248755310181)) ;
#79681=CARTESIAN_POINT('',(129.131255473727,-76.1306363338479,-197.312255310181)) ;
#79682=CARTESIAN_POINT('Ctrl Pts',(129.032653559991,-76.1941363338485,-197.24875531018)) ;
#79683=CARTESIAN_POINT('Ctrl Pts',(129.039651623408,-76.1883808250969,-197.24875531018)) ;
#79684=CARTESIAN_POINT('Ctrl Pts',(129.046266473008,-76.1820606916736,-197.24953905352)) ;
#79685=CARTESIAN_POINT('Ctrl Pts',(129.064384732645,-76.1646337439627,-197.254884983357)) ;
#79686=CARTESIAN_POINT('Ctrl Pts',(129.075133233964,-76.1543405140722,-197.261267814065)) ;
#79687=CARTESIAN_POINT('Ctrl Pts',(129.094006424647,-76.1413439673982,-197.276182188303)) ;
#79688=CARTESIAN_POINT('Ctrl Pts',(129.101141169816,-76.1374914691481,-197.282617198857)) ;
#79689=CARTESIAN_POINT('Ctrl Pts',(129.115569600563,-76.1322072351016,-197.296404775943)) ;
#79690=CARTESIAN_POINT('Ctrl Pts',(129.122766847883,-76.130795216541,-197.303665859274)) ;
#79691=CARTESIAN_POINT('Ctrl Pts',(129.13042019884,-76.1306405541772,-197.311409957671)) ;
#79692=CARTESIAN_POINT('Ctrl Pts',(129.130837836329,-76.1306363338479,-197.311832627557)) ;
#79693=CARTESIAN_POINT('Ctrl Pts',(129.131255473728,-76.1306363338479,-197.31225531018)) ;
#79694=CARTESIAN_POINT('',(126.238286869423,-76.1306363338479,-197.31225531018)) ;
#79695=CARTESIAN_POINT('Origin',(126.238286869421,-76.194136333848,-204.48775531018)) ;
#79696=CARTESIAN_POINT('',(132.552818265116,-76.1306363338479,-204.487755310181)) ;
#79697=CARTESIAN_POINT('Ctrl Pts',(132.651420178853,-76.1941363338479,-204.551255310181)) ;
#79698=CARTESIAN_POINT('Ctrl Pts',(132.644422115437,-76.1883808250966,-204.551255310181)) ;
#79699=CARTESIAN_POINT('Ctrl Pts',(132.637807265836,-76.1820606916732,-204.550471566842)) ;
#79700=CARTESIAN_POINT('Ctrl Pts',(132.619689006197,-76.1646337439608,-204.545125637004)) ;
#79701=CARTESIAN_POINT('Ctrl Pts',(132.608940504879,-76.1543405140707,-204.538742806295)) ;
#79702=CARTESIAN_POINT('Ctrl Pts',(132.590067314197,-76.1413439673978,-204.523828432057)) ;
#79703=CARTESIAN_POINT('Ctrl Pts',(132.582932569028,-76.1374914691479,-204.517393421504)) ;
#79704=CARTESIAN_POINT('Ctrl Pts',(132.568504138281,-76.1322072351013,-204.503605844418)) ;
#79705=CARTESIAN_POINT('Ctrl Pts',(132.561306890966,-76.1307952165411,-204.496344761088)) ;
#79706=CARTESIAN_POINT('Ctrl Pts',(132.553653540003,-76.1306405541772,-204.48860066269)) ;
#79707=CARTESIAN_POINT('Ctrl Pts',(132.553235902516,-76.1306363338479,-204.488177992805)) ;
#79708=CARTESIAN_POINT('Ctrl Pts',(132.552818265117,-76.1306363338479,-204.487755310181)) ;
#79709=CARTESIAN_POINT('',(129.131255473726,-76.1306363338479,-204.487755310181)) ;
#79710=CARTESIAN_POINT('',(126.238286869421,-76.1306363338479,-204.48775531018)) ;
#79711=CARTESIAN_POINT('Ctrl Pts',(129.131255473726,-76.1306363338479,-204.487755310181)) ;
#79712=CARTESIAN_POINT('Ctrl Pts',(129.130837836326,-76.1306363338479,-204.488177992804)) ;
#79713=CARTESIAN_POINT('Ctrl Pts',(129.130420198838,-76.1306405541772,-204.48860066269)) ;
#79714=CARTESIAN_POINT('Ctrl Pts',(129.122766847881,-76.1307952165411,-204.496344761087)) ;
#79715=CARTESIAN_POINT('Ctrl Pts',(129.115569600561,-76.1322072351016,-204.503605844418)) ;
#79716=CARTESIAN_POINT('Ctrl Pts',(129.101141169815,-76.1374914691477,-204.517393421503)) ;
#79717=CARTESIAN_POINT('Ctrl Pts',(129.094006424646,-76.1413439673975,-204.523828432056)) ;
#79718=CARTESIAN_POINT('Ctrl Pts',(129.075133233963,-76.1543405140709,-204.538742806295)) ;
#79719=CARTESIAN_POINT('Ctrl Pts',(129.064384732644,-76.1646337439613,-204.545125637003)) ;
#79720=CARTESIAN_POINT('Ctrl Pts',(129.046266473007,-76.1820606916719,-204.550471566841)) ;
#79721=CARTESIAN_POINT('Ctrl Pts',(129.039651623407,-76.1883808250955,-204.55125531018)) ;
#79722=CARTESIAN_POINT('Ctrl Pts',(129.03265355999,-76.1941363338474,-204.55125531018)) ;
#79723=CARTESIAN_POINT('Origin',(132.842036869421,-75.178136333848,-209.631255310181)) ;
#79724=CARTESIAN_POINT('',(132.842036869423,-80.3871363338479,-197.123755310181)) ;
#79725=CARTESIAN_POINT('',(132.842036869423,-80.3871363338479,-196.421255310181)) ;
#79726=CARTESIAN_POINT('',(132.842036869422,-80.3871363338479,-199.185505310181)) ;
#79727=CARTESIAN_POINT('',(132.842036869423,-76.2556363338479,-197.123755310181)) ;
#79728=CARTESIAN_POINT('',(132.842036869423,-79.7183863338479,-197.123755310181)) ;
#79729=CARTESIAN_POINT('',(132.842036869423,-76.2556363338479,-196.421255310181)) ;
#79730=CARTESIAN_POINT('',(132.842036869421,-76.2556363338479,-205.265630310181)) ;
#79731=CARTESIAN_POINT('',(132.842036869423,-74.8923863338479,-196.421255310181)) ;
#79732=CARTESIAN_POINT('Origin',(132.717036869423,-79.7183863338479,-197.123755310181)) ;
#79733=CARTESIAN_POINT('Origin',(132.717036869423,-80.3871363338479,-197.123755310181)) ;
#79734=CARTESIAN_POINT('Origin',(132.717036869423,-76.2556363338479,-197.123755310181)) ;
#79735=CARTESIAN_POINT('Origin',(134.84203686942,-75.1781363338479,-209.631255310181)) ;
#79736=CARTESIAN_POINT('',(134.842036869421,-76.0056363338479,-205.378755310181)) ;
#79737=CARTESIAN_POINT('',(134.842036869422,-76.0056363338479,-196.421255310181)) ;
#79738=CARTESIAN_POINT('',(134.842036869421,-76.0056363338479,-205.265630310181)) ;
#79739=CARTESIAN_POINT('',(134.842036869421,-75.8766363338479,-205.378755310181)) ;
#79740=CARTESIAN_POINT('',(134.842036869421,-79.7183863338479,-205.378755310181)) ;
#79741=CARTESIAN_POINT('',(134.842036869421,-75.3031363338479,-204.805255310181)) ;
#79742=CARTESIAN_POINT('Origin',(134.842036869421,-75.8766363338479,-204.805255310181)) ;
#79743=CARTESIAN_POINT('',(134.842036869422,-75.3031363338479,-196.994755310181)) ;
#79744=CARTESIAN_POINT('',(134.842036869421,-75.3031363338479,-205.265630310181)) ;
#79745=CARTESIAN_POINT('',(134.842036869422,-75.8766363338479,-196.421255310181)) ;
#79746=CARTESIAN_POINT('Origin',(134.842036869422,-75.8766363338479,-196.994755310181)) ;
#79747=CARTESIAN_POINT('',(134.842036869422,-74.8923863338479,-196.421255310181)) ;
#79748=CARTESIAN_POINT('Origin',(126.842036869421,-79.115506191122,-200.900107016444)) ;
#79749=CARTESIAN_POINT('',(126.842036869422,-75.8766363338479,-196.42125531018)) ;
#79750=CARTESIAN_POINT('',(126.842036869422,-76.0056363338479,-196.42125531018)) ;
#79751=CARTESIAN_POINT('',(126.842036869422,-76.8610712624849,-196.42125531018)) ;
#79752=CARTESIAN_POINT('',(126.842036869421,-75.3031363338479,-196.99475531018)) ;
#79753=CARTESIAN_POINT('Origin',(126.842036869421,-75.8766363338479,-196.99475531018)) ;
#79754=CARTESIAN_POINT('',(126.84203686942,-75.3031363338479,-204.80525531018)) ;
#79755=CARTESIAN_POINT('',(126.842036869421,-75.3031363338479,-200.900056163312)) ;
#79756=CARTESIAN_POINT('',(126.84203686942,-75.8766363338479,-205.37875531018)) ;
#79757=CARTESIAN_POINT('Origin',(126.84203686942,-75.8766363338479,-204.80525531018)) ;
#79758=CARTESIAN_POINT('',(126.84203686942,-76.0056363338479,-205.37875531018)) ;
#79759=CARTESIAN_POINT('',(126.84203686942,-81.6870712624849,-205.37875531018)) ;
#79760=CARTESIAN_POINT('',(126.842036869421,-76.0056363338479,-200.900056163312)) ;
#79761=CARTESIAN_POINT('Origin',(128.967036869422,-81.687071262485,-197.123755310181)) ;
#79762=CARTESIAN_POINT('',(128.842036869422,-80.3871363338479,-197.123755310181)) ;
#79763=CARTESIAN_POINT('Origin',(128.967036869422,-80.3871363338479,-197.123755310181)) ;
#79764=CARTESIAN_POINT('',(128.842036869422,-76.2556363338479,-197.123755310181)) ;
#79765=CARTESIAN_POINT('',(128.842036869422,-81.687071262485,-197.123755310181)) ;
#79766=CARTESIAN_POINT('Origin',(128.967036869422,-76.2556363338479,-197.123755310181)) ;
#79767=CARTESIAN_POINT('Origin',(128.842036869421,-79.1155061911221,-200.900107016445)) ;
#79768=CARTESIAN_POINT('',(128.842036869422,-80.3871363338479,-196.42125531018)) ;
#79769=CARTESIAN_POINT('',(128.842036869422,-80.3871363338479,-194.819931163313)) ;
#79770=CARTESIAN_POINT('',(128.842036869422,-76.2556363338479,-196.42125531018)) ;
#79771=CARTESIAN_POINT('',(128.842036869422,-76.861071262485,-196.42125531018)) ;
#79772=CARTESIAN_POINT('',(128.842036869421,-76.2556363338479,-200.900056163313)) ;
#79773=CARTESIAN_POINT('Origin',(132.717036869422,-76.2556363338479,-204.676255310181)) ;
#79774=CARTESIAN_POINT('',(132.967036869422,-76.1306363338479,-204.676255310181)) ;
#79775=CARTESIAN_POINT('Origin',(132.967036869422,-76.2556363338479,-204.676255310181)) ;
#79776=CARTESIAN_POINT('Origin',(132.717036869422,-76.1306363338479,-204.676255310181)) ;
#79777=CARTESIAN_POINT('Origin',(128.967036869421,-76.2556363338479,-204.676255310181)) ;
#79778=CARTESIAN_POINT('',(128.717036869421,-76.1306363338479,-204.676255310181)) ;
#79779=CARTESIAN_POINT('Origin',(128.967036869421,-76.1306363338479,-204.676255310181)) ;
#79780=CARTESIAN_POINT('Origin',(128.717036869421,-76.2556363338479,-204.676255310181)) ;
#79781=CARTESIAN_POINT('Origin',(132.717036869423,-76.2556363338479,-197.123755310181)) ;
#79782=CARTESIAN_POINT('',(132.967036869423,-76.1306363338479,-197.123755310181)) ;
#79783=CARTESIAN_POINT('Origin',(132.717036869423,-76.1306363338479,-197.123755310181)) ;
#79784=CARTESIAN_POINT('Origin',(132.967036869423,-76.2556363338479,-197.123755310181)) ;
#79785=CARTESIAN_POINT('Origin',(128.967036869422,-80.3871363338479,-197.123755310181)) ;
#79786=CARTESIAN_POINT('Origin',(128.967036869422,-80.3871363338479,-197.123755310181)) ;
#79787=CARTESIAN_POINT('Origin',(128.967036869422,-80.3871363338479,-197.123755310181)) ;
#79788=CARTESIAN_POINT('Origin',(128.967036869422,-76.2556363338479,-197.123755310181)) ;
#79789=CARTESIAN_POINT('',(128.717036869422,-76.1306363338479,-197.123755310181)) ;
#79790=CARTESIAN_POINT('Origin',(128.717036869422,-76.2556363338479,-197.123755310181)) ;
#79791=CARTESIAN_POINT('Origin',(128.967036869422,-76.1306363338479,-197.123755310181)) ;
#79792=CARTESIAN_POINT('Origin',(132.717036869423,-80.3871363338479,-197.123755310181)) ;
#79793=CARTESIAN_POINT('Origin',(132.717036869423,-80.3871363338479,-197.123755310181)) ;
#79794=CARTESIAN_POINT('Origin',(132.717036869423,-80.3871363338479,-197.123755310181)) ;
#79795=CARTESIAN_POINT('Origin',(128.857661869423,-80.3871363338479,-197.123755310181)) ;
#79796=CARTESIAN_POINT('Origin',(132.967036869421,-76.2556363338479,-205.265630310181)) ;
#79797=CARTESIAN_POINT('',(132.967036869421,-76.1306363338479,-205.378755310181)) ;
#79798=CARTESIAN_POINT('Origin',(132.967036869421,-76.2556363338479,-205.378755310181)) ;
#79799=CARTESIAN_POINT('',(132.967036869421,-76.1306363338479,-205.265630310181)) ;
#79800=CARTESIAN_POINT('Origin',(128.717036869421,-76.2556363338479,-200.900056163313)) ;
#79801=CARTESIAN_POINT('',(128.717036869421,-76.1306363338479,-205.37875531018)) ;
#79802=CARTESIAN_POINT('',(128.717036869421,-76.1306363338479,-200.900056163313)) ;
#79803=CARTESIAN_POINT('Origin',(128.717036869421,-76.2556363338479,-205.37875531018)) ;
#79804=CARTESIAN_POINT('Origin',(126.238286869421,-76.0056363338479,-205.37875531018)) ;
#79805=CARTESIAN_POINT('',(134.717036869421,-76.1306363338479,-205.378755310181)) ;
#79806=CARTESIAN_POINT('Origin',(134.717036869421,-76.0056363338479,-205.378755310181)) ;
#79807=CARTESIAN_POINT('',(126.238286869421,-76.1306363338479,-205.37875531018)) ;
#79808=CARTESIAN_POINT('Origin',(132.967036869421,-76.0056363338479,-205.378755310181)) ;
#79809=CARTESIAN_POINT('Origin',(126.238286869421,-76.0056363338479,-205.37875531018)) ;
#79810=CARTESIAN_POINT('Origin',(128.717036869421,-76.0056363338479,-205.37875531018)) ;
#79811=CARTESIAN_POINT('',(126.96703686942,-76.1306363338479,-205.37875531018)) ;
#79812=CARTESIAN_POINT('',(126.238286869421,-76.1306363338479,-205.37875531018)) ;
#79813=CARTESIAN_POINT('Origin',(126.96703686942,-76.0056363338479,-205.37875531018)) ;
#79814=CARTESIAN_POINT('Origin',(134.717036869422,-74.8923863338479,-196.421255310181)) ;
#79815=CARTESIAN_POINT('Origin',(134.717036869422,-76.0056363338479,-196.421255310181)) ;
#79816=CARTESIAN_POINT('Origin',(134.717036869422,-75.8766363338479,-196.421255310181)) ;
#79817=CARTESIAN_POINT('Origin',(134.717036869422,-75.8766363338479,-196.994755310181)) ;
#79818=CARTESIAN_POINT('Origin',(134.717036869422,-75.3031363338479,-196.994755310181)) ;
#79819=CARTESIAN_POINT('Origin',(134.717036869421,-75.3031363338479,-205.265630310181)) ;
#79820=CARTESIAN_POINT('Origin',(134.717036869421,-75.3031363338479,-204.805255310181)) ;
#79821=CARTESIAN_POINT('Origin',(134.717036869421,-75.8766363338479,-204.805255310181)) ;
#79822=CARTESIAN_POINT('Origin',(134.717036869421,-75.8766363338479,-205.378755310181)) ;
#79823=CARTESIAN_POINT('Origin',(134.717036869421,-79.7183863338479,-205.378755310181)) ;
#79824=CARTESIAN_POINT('Origin',(134.717036869421,-76.0056363338479,-205.378755310181)) ;
#79825=CARTESIAN_POINT('Origin',(134.717036869421,-76.0056363338479,-205.265630310181)) ;
#79826=CARTESIAN_POINT('',(134.717036869422,-76.1306363338479,-196.421255310181)) ;
#79827=CARTESIAN_POINT('Origin',(134.717036869422,-76.0056363338479,-196.421255310181)) ;
#79828=CARTESIAN_POINT('',(134.717036869421,-76.1306363338479,-205.265630310181)) ;
#79829=CARTESIAN_POINT('Origin',(134.717036869421,-76.0056363338479,-205.378755310181)) ;
#79830=CARTESIAN_POINT('Origin',(126.967036869421,-76.0056363338479,-200.900056163312)) ;
#79831=CARTESIAN_POINT('Origin',(126.96703686942,-76.0056363338479,-205.37875531018)) ;
#79832=CARTESIAN_POINT('',(126.967036869422,-76.1306363338479,-196.42125531018)) ;
#79833=CARTESIAN_POINT('',(126.967036869421,-76.1306363338479,-200.900056163312)) ;
#79834=CARTESIAN_POINT('Origin',(126.967036869422,-76.0056363338479,-196.42125531018)) ;
#79835=CARTESIAN_POINT('Origin',(126.96703686942,-81.6870712624849,-205.37875531018)) ;
#79836=CARTESIAN_POINT('Origin',(126.96703686942,-76.0056363338479,-205.37875531018)) ;
#79837=CARTESIAN_POINT('Origin',(126.96703686942,-75.8766363338479,-205.37875531018)) ;
#79838=CARTESIAN_POINT('Origin',(126.96703686942,-75.8766363338479,-204.80525531018)) ;
#79839=CARTESIAN_POINT('Origin',(126.96703686942,-75.3031363338479,-204.80525531018)) ;
#79840=CARTESIAN_POINT('Origin',(126.967036869421,-75.3031363338479,-200.900056163312)) ;
#79841=CARTESIAN_POINT('Origin',(126.967036869421,-75.3031363338479,-196.99475531018)) ;
#79842=CARTESIAN_POINT('Origin',(126.967036869421,-75.8766363338479,-196.99475531018)) ;
#79843=CARTESIAN_POINT('Origin',(126.967036869422,-75.8766363338479,-196.42125531018)) ;
#79844=CARTESIAN_POINT('Origin',(126.967036869422,-76.8610712624849,-196.42125531018)) ;
#79845=CARTESIAN_POINT('Origin',(126.967036869422,-76.0056363338479,-196.42125531018)) ;
#79846=CARTESIAN_POINT('Origin',(132.967036869421,-76.2556363338479,-205.265630310181)) ;
#79847=CARTESIAN_POINT('',(132.967036869423,-76.1306363338479,-196.421255310181)) ;
#79848=CARTESIAN_POINT('',(132.967036869421,-76.1306363338479,-205.265630310181)) ;
#79849=CARTESIAN_POINT('Origin',(132.967036869423,-76.2556363338479,-196.421255310181)) ;
#79850=CARTESIAN_POINT('Origin',(132.717036869423,-74.8923863338479,-196.421255310181)) ;
#79851=CARTESIAN_POINT('Origin',(132.717036869423,-80.3871363338479,-196.421255310181)) ;
#79852=CARTESIAN_POINT('Origin',(132.717036869423,-76.2556363338479,-196.421255310181)) ;
#79853=CARTESIAN_POINT('Origin',(132.717036869422,-80.3871363338479,-199.185505310181)) ;
#79854=CARTESIAN_POINT('Origin',(132.717036869423,-80.3871363338479,-196.421255310181)) ;
#79855=CARTESIAN_POINT('Origin',(128.967036869422,-80.3871363338479,-194.819931163313)) ;
#79856=CARTESIAN_POINT('Origin',(128.967036869422,-80.3871363338479,-196.42125531018)) ;
#79857=CARTESIAN_POINT('Origin',(128.967036869422,-76.861071262485,-196.42125531018)) ;
#79858=CARTESIAN_POINT('Origin',(128.967036869422,-76.2556363338479,-196.42125531018)) ;
#79859=CARTESIAN_POINT('Origin',(128.967036869422,-80.3871363338479,-196.42125531018)) ;
#79860=CARTESIAN_POINT('Origin',(128.857661869422,-80.3871363338479,-196.42125531018)) ;
#79861=CARTESIAN_POINT('Origin',(132.717036869423,-80.3871363338479,-196.421255310181)) ;
#79862=CARTESIAN_POINT('Origin',(128.967036869422,-80.3871363338479,-196.42125531018)) ;
#79863=CARTESIAN_POINT('Origin',(128.967036869422,-80.3871363338479,-196.42125531018)) ;
#79864=CARTESIAN_POINT('Origin',(132.717036869423,-80.3871363338479,-196.421255310181)) ;
#79865=CARTESIAN_POINT('Origin',(128.717036869421,-76.2556363338479,-200.900056163313)) ;
#79866=CARTESIAN_POINT('',(128.717036869422,-76.1306363338479,-196.42125531018)) ;
#79867=CARTESIAN_POINT('Origin',(128.717036869422,-76.2556363338479,-196.42125531018)) ;
#79868=CARTESIAN_POINT('',(128.717036869421,-76.1306363338479,-200.900056163313)) ;
#79869=CARTESIAN_POINT('Origin',(126.238286869422,-76.0056363338479,-196.42125531018)) ;
#79870=CARTESIAN_POINT('Origin',(126.967036869422,-76.0056363338479,-196.42125531018)) ;
#79871=CARTESIAN_POINT('',(126.238286869422,-76.1306363338479,-196.42125531018)) ;
#79872=CARTESIAN_POINT('Origin',(128.717036869422,-76.0056363338479,-196.42125531018)) ;
#79873=CARTESIAN_POINT('Origin',(128.717036869422,-76.2556363338479,-196.42125531018)) ;
#79874=CARTESIAN_POINT('Origin',(126.238286869422,-76.0056363338479,-196.42125531018)) ;
#79875=CARTESIAN_POINT('Origin',(132.967036869423,-76.0056363338479,-196.421255310181)) ;
#79876=CARTESIAN_POINT('',(126.238286869422,-76.1306363338479,-196.42125531018)) ;
#79877=CARTESIAN_POINT('Origin',(134.717036869422,-76.0056363338479,-196.421255310181)) ;
#79878=CARTESIAN_POINT('Origin',(132.967036869423,-76.2556363338479,-196.421255310181)) ;
#79879=CARTESIAN_POINT('Origin',(126.967036869422,-76.0056363338479,-196.42125531018)) ;
#79880=CARTESIAN_POINT('Origin',(134.717036869422,-76.0056363338479,-196.421255310181)) ;
#79881=CARTESIAN_POINT('Origin',(126.96703686942,-76.0056363338479,-205.37875531018)) ;
#79882=CARTESIAN_POINT('Origin',(134.717036869421,-76.0056363338479,-205.378755310181)) ;
#79883=CARTESIAN_POINT('Origin',(128.717036869421,-76.2556363338479,-205.37875531018)) ;
#79884=CARTESIAN_POINT('Origin',(132.967036869421,-76.2556363338479,-205.378755310181)) ;
#79885=CARTESIAN_POINT('Origin',(130.842036869422,-78.037636333848,-200.900005310181)) ;
#79886=CARTESIAN_POINT('',(130.842036869423,-78.162636333848,-198.167505310181)) ;
#79887=CARTESIAN_POINT('Origin',(130.842036869422,-78.162636333848,-200.900005310181)) ;
#79888=CARTESIAN_POINT('',(130.842036869423,-78.037636333848,-198.042505310181)) ;
#79889=CARTESIAN_POINT('Origin',(130.842036869422,-78.037636333848,-198.167505310181)) ;
#79890=CARTESIAN_POINT('Origin',(130.842036869422,-78.037636333848,-200.900005310181)) ;
#79891=CARTESIAN_POINT('Origin',(126.238286869422,-76.1306363338479,-200.90000531018)) ;
#79892=CARTESIAN_POINT('',(130.842036869422,-76.1306363338479,-203.882505310181)) ;
#79893=CARTESIAN_POINT('Origin',(130.842036869422,-76.1306363338479,-200.900005310181)) ;
#79894=CARTESIAN_POINT('Origin',(130.842036869422,-76.130636333848,-200.900005310181)) ;
#79895=CARTESIAN_POINT('',(130.842036869422,-76.2556363338479,-203.757505310181)) ;
#79896=CARTESIAN_POINT('',(130.842036869422,-76.2556363338479,-198.042505310181)) ;
#79897=CARTESIAN_POINT('Origin',(130.842036869422,-76.2556363338479,-200.900005310181)) ;
#79898=CARTESIAN_POINT('Origin',(130.842036869422,-76.2556363338479,-200.900005310181)) ;
#79899=CARTESIAN_POINT('',(130.842036869422,-76.130636333848,-198.042505310181)) ;
#79900=CARTESIAN_POINT('Origin',(130.842036869422,-76.2556363338479,-200.900005310181)) ;
#79901=CARTESIAN_POINT('Origin',(130.842036869422,-76.2556363338479,-203.882505310181)) ;
#79902=CARTESIAN_POINT('Origin',(134.413911869422,-78.162636333848,-204.471880310181)) ;
#79903=CARTESIAN_POINT('Ctrl Pts',(130.148682626495,-78.162636333848,-199.569870018636)) ;
#79904=CARTESIAN_POINT('Ctrl Pts',(130.287989560911,-78.162636333848,-199.468610877589)) ;
#79905=CARTESIAN_POINT('Ctrl Pts',(130.443609984945,-78.162636333848,-199.392079607406)) ;
#79906=CARTESIAN_POINT('Ctrl Pts',(130.818610624952,-78.162636333848,-199.281692556162)) ;
#79907=CARTESIAN_POINT('Ctrl Pts',(131.013241952139,-78.162636333848,-199.274293448841)) ;
#79908=CARTESIAN_POINT('Ctrl Pts',(131.29629180081,-78.162636333848,-199.292439790627)) ;
#79909=CARTESIAN_POINT('Ctrl Pts',(131.426707517184,-78.162636333848,-199.316460614013)) ;
#79910=CARTESIAN_POINT('Ctrl Pts',(131.684331081807,-78.162636333848,-199.396206322493)) ;
#79911=CARTESIAN_POINT('Ctrl Pts',(131.810182908812,-78.162636333848,-199.452859887612)) ;
#79912=CARTESIAN_POINT('Ctrl Pts',(131.927746211475,-78.162636333848,-199.52419935635)) ;
#79913=CARTESIAN_POINT('Ctrl Pts',(132.582591006102,-78.162636333848,-200.694875936258)) ;
#79914=CARTESIAN_POINT('Ctrl Pts',(132.581738268888,-78.162636333848,-200.854045453659)) ;
#79915=CARTESIAN_POINT('Ctrl Pts',(132.560263297441,-78.162636333848,-201.03274583285)) ;
#79916=CARTESIAN_POINT('Ctrl Pts',(132.446670912049,-78.162636333848,-201.375601546739)) ;
#79917=CARTESIAN_POINT('Ctrl Pts',(132.371376067505,-78.1626363339111,-201.523340523348)) ;
#79918=CARTESIAN_POINT('Ctrl Pts',(132.188297852137,-78.1626363339111,-201.778075291675)) ;
#79919=CARTESIAN_POINT('Ctrl Pts',(132.085318536322,-78.162636333848,-201.886377279636)) ;
#79920=CARTESIAN_POINT('Ctrl Pts',(131.895362496131,-78.162636333848,-202.038032714918)) ;
#79921=CARTESIAN_POINT('Ctrl Pts',(131.770997671067,-78.162636333848,-202.126855902566)) ;
#79922=CARTESIAN_POINT('Ctrl Pts',(131.596354821607,-78.162636333848,-202.196540858098)) ;
#79923=CARTESIAN_POINT('Ctrl Pts',(135.341831707641,-78.9434337333926,-200.900005310181)) ;
#79924=CARTESIAN_POINT('Ctrl Pts',(135.341831707641,-78.8938243583926,-202.763881360068)) ;
#79925=CARTESIAN_POINT('Ctrl Pts',(134.023872313475,-78.8442149833926,-204.081840754234)) ;
#79926=CARTESIAN_POINT('Ctrl Pts',(132.705912919309,-78.7946056083926,-205.3998001484)) ;
#79927=CARTESIAN_POINT('Ctrl Pts',(130.842036869423,-78.7449962333926,-205.3998001484)) ;
#79928=CARTESIAN_POINT('Ctrl Pts',(128.978160819536,-78.6953868583926,-205.3998001484)) ;
#79929=CARTESIAN_POINT('Ctrl Pts',(127.66020142537,-78.6457774833926,-204.081840754234)) ;
#79930=CARTESIAN_POINT('Ctrl Pts',(126.342242031204,-78.5961681083926,-202.763881360068)) ;
#79931=CARTESIAN_POINT('Ctrl Pts',(126.342242031204,-78.5465587333926,-200.900005310181)) ;
#79932=CARTESIAN_POINT('Ctrl Pts',(126.342242031204,-78.4969493583926,-199.036129260295)) ;
#79933=CARTESIAN_POINT('Ctrl Pts',(127.66020142537,-78.4473399833926,-197.718169866129)) ;
#79934=CARTESIAN_POINT('Ctrl Pts',(128.978160819536,-78.3977306083926,-196.400210471963)) ;
#79935=CARTESIAN_POINT('Ctrl Pts',(130.842036869422,-78.3481212333926,-196.400210471963)) ;
#79936=CARTESIAN_POINT('Ctrl Pts',(132.705912919309,-78.2985118583926,-196.400210471962)) ;
#79937=CARTESIAN_POINT('Ctrl Pts',(134.023872313475,-78.2489024833926,-197.718169866128)) ;
#79938=CARTESIAN_POINT('Ctrl Pts',(135.341831707641,-78.1992931083926,-199.036129260294)) ;
#79939=CARTESIAN_POINT('Ctrl Pts',(135.341831707641,-78.1496837333926,-200.900005310181)) ;
#79940=CARTESIAN_POINT('Ctrl Pts',(135.341831707641,-78.1000743583926,-202.763881360068)) ;
#79941=CARTESIAN_POINT('Ctrl Pts',(134.023872313475,-78.0504649833926,-204.081840754234)) ;
#79942=CARTESIAN_POINT('Ctrl Pts',(132.705912919309,-78.0008556083926,-205.3998001484)) ;
#79943=CARTESIAN_POINT('Ctrl Pts',(130.842036869423,-77.9512462333926,-205.3998001484)) ;
#79944=CARTESIAN_POINT('Ctrl Pts',(128.978160819536,-77.9016368583926,-205.3998001484)) ;
#79945=CARTESIAN_POINT('Ctrl Pts',(127.66020142537,-77.8520274833926,-204.081840754234)) ;
#79946=CARTESIAN_POINT('Ctrl Pts',(126.342242031204,-77.8024181083926,-202.763881360068)) ;
#79947=CARTESIAN_POINT('Ctrl Pts',(126.342242031204,-77.7528087333926,-200.900005310181)) ;
#79948=CARTESIAN_POINT('Ctrl Pts',(126.342242031204,-77.7031993583927,-199.036129260295)) ;
#79949=CARTESIAN_POINT('Ctrl Pts',(127.66020142537,-77.6535899833926,-197.718169866129)) ;
#79950=CARTESIAN_POINT('Ctrl Pts',(128.978160819536,-77.6039806083926,-196.400210471963)) ;
#79951=CARTESIAN_POINT('Ctrl Pts',(130.842036869422,-77.5543712333926,-196.400210471963)) ;
#79952=CARTESIAN_POINT('Ctrl Pts',(132.705912919309,-77.5047618583926,-196.400210471962)) ;
#79953=CARTESIAN_POINT('Ctrl Pts',(134.023872313475,-77.4551524833926,-197.718169866128)) ;
#79954=CARTESIAN_POINT('Ctrl Pts',(135.341831707641,-77.4055431083926,-199.036129260294)) ;
#79955=CARTESIAN_POINT('Ctrl Pts',(135.341831707641,-77.3559337333926,-200.900005310181)) ;
#79956=CARTESIAN_POINT('Ctrl Pts',(135.341831707641,-77.3063243583926,-202.763881360068)) ;
#79957=CARTESIAN_POINT('Ctrl Pts',(134.023872313475,-77.2567149833926,-204.081840754234)) ;
#79958=CARTESIAN_POINT('Ctrl Pts',(132.705912919309,-77.2071056083926,-205.3998001484)) ;
#79959=CARTESIAN_POINT('Ctrl Pts',(130.842036869423,-77.1574962333926,-205.3998001484)) ;
#79960=CARTESIAN_POINT('Ctrl Pts',(128.978160819536,-77.1078868583926,-205.3998001484)) ;
#79961=CARTESIAN_POINT('Ctrl Pts',(127.66020142537,-77.0582774833926,-204.081840754234)) ;
#79962=CARTESIAN_POINT('Ctrl Pts',(126.342242031204,-77.0086681083926,-202.763881360068)) ;
#79963=CARTESIAN_POINT('Ctrl Pts',(126.342242031204,-76.9590587333926,-200.900005310181)) ;
#79964=CARTESIAN_POINT('Ctrl Pts',(126.342242031204,-76.9094493583926,-199.036129260295)) ;
#79965=CARTESIAN_POINT('Ctrl Pts',(127.66020142537,-76.8598399833926,-197.718169866129)) ;
#79966=CARTESIAN_POINT('Ctrl Pts',(128.978160819536,-76.8102306083926,-196.400210471963)) ;
#79967=CARTESIAN_POINT('Ctrl Pts',(130.842036869422,-76.7606212333926,-196.400210471963)) ;
#79968=CARTESIAN_POINT('Ctrl Pts',(132.705912919309,-76.7110118583926,-196.400210471962)) ;
#79969=CARTESIAN_POINT('Ctrl Pts',(134.023872313475,-76.6614024833926,-197.718169866128)) ;
#79970=CARTESIAN_POINT('Ctrl Pts',(135.341831707641,-76.6117931083926,-199.036129260294)) ;
#79971=CARTESIAN_POINT('Ctrl Pts',(135.341831707641,-76.5621837333926,-200.900005310181)) ;
#79972=CARTESIAN_POINT('Ctrl Pts',(135.341831707641,-76.5125743583926,-202.763881360068)) ;
#79973=CARTESIAN_POINT('Ctrl Pts',(134.023872313475,-76.4629649833926,-204.081840754234)) ;
#79974=CARTESIAN_POINT('Ctrl Pts',(132.705912919309,-76.4133556083926,-205.3998001484)) ;
#79975=CARTESIAN_POINT('Ctrl Pts',(130.842036869423,-76.3637462333926,-205.3998001484)) ;
#79976=CARTESIAN_POINT('Ctrl Pts',(128.978160819536,-76.3141368583926,-205.3998001484)) ;
#79977=CARTESIAN_POINT('Ctrl Pts',(127.66020142537,-76.2645274833926,-204.081840754234)) ;
#79978=CARTESIAN_POINT('Ctrl Pts',(126.342242031204,-76.2149181083926,-202.763881360068)) ;
#79979=CARTESIAN_POINT('Ctrl Pts',(126.342242031204,-76.1653087333926,-200.900005310181)) ;
#79980=CARTESIAN_POINT('Ctrl Pts',(126.342242031204,-76.1156993583926,-199.036129260295)) ;
#79981=CARTESIAN_POINT('Ctrl Pts',(127.66020142537,-76.0660899833926,-197.718169866129)) ;
#79982=CARTESIAN_POINT('Ctrl Pts',(128.978160819536,-76.0164806083926,-196.400210471963)) ;
#79983=CARTESIAN_POINT('Ctrl Pts',(130.842036869422,-75.9668712333926,-196.400210471963)) ;
#79984=CARTESIAN_POINT('Ctrl Pts',(132.705912919309,-75.9172618583926,-196.400210471962)) ;
#79985=CARTESIAN_POINT('Ctrl Pts',(134.023872313475,-75.8676524833926,-197.718169866128)) ;
#79986=CARTESIAN_POINT('Ctrl Pts',(135.341831707641,-75.8180431083926,-199.036129260294)) ;
#79987=CARTESIAN_POINT('Ctrl Pts',(135.341831707641,-75.7684337333926,-200.900005310181)) ;
#79988=CARTESIAN_POINT('Ctrl Pts',(135.341831707641,-75.7188243583926,-202.763881360068)) ;
#79989=CARTESIAN_POINT('Ctrl Pts',(134.023872313475,-75.6692149833926,-204.081840754234)) ;
#79990=CARTESIAN_POINT('Ctrl Pts',(132.705912919309,-75.6196056083926,-205.3998001484)) ;
#79991=CARTESIAN_POINT('Ctrl Pts',(130.842036869422,-75.5699962333926,-205.3998001484)) ;
#79992=CARTESIAN_POINT('Ctrl Pts',(128.978160819536,-75.5203868583926,-205.3998001484)) ;
#79993=CARTESIAN_POINT('Ctrl Pts',(127.66020142537,-75.4707774833926,-204.081840754234)) ;
#79994=CARTESIAN_POINT('Ctrl Pts',(126.342242031204,-75.4211681083926,-202.763881360068)) ;
#79995=CARTESIAN_POINT('Ctrl Pts',(126.342242031204,-75.3715587333926,-200.900005310181)) ;
#79996=CARTESIAN_POINT('Ctrl Pts',(126.342242031204,-75.3219493583926,-199.036129260295)) ;
#79997=CARTESIAN_POINT('Ctrl Pts',(127.66020142537,-75.2723399833926,-197.718169866129)) ;
#79998=CARTESIAN_POINT('Ctrl Pts',(128.978160819536,-75.2227306083926,-196.400210471963)) ;
#79999=CARTESIAN_POINT('Ctrl Pts',(130.842036869422,-75.1731212333926,-196.400210471963)) ;
#80000=CARTESIAN_POINT('Ctrl Pts',(132.705912919309,-75.1235118583926,-196.400210471962)) ;
#80001=CARTESIAN_POINT('Ctrl Pts',(134.023872313475,-75.0739024833926,-197.718169866128)) ;
#80002=CARTESIAN_POINT('Ctrl Pts',(135.341831707641,-75.0242931083926,-199.036129260294)) ;
#80003=CARTESIAN_POINT('Ctrl Pts',(135.341831707641,-74.9746837333926,-200.900005310181)) ;
#80004=CARTESIAN_POINT('Ctrl Pts',(135.341831707641,-74.9250743583926,-202.763881360068)) ;
#80005=CARTESIAN_POINT('Ctrl Pts',(134.023872313475,-74.8754649833926,-204.081840754234)) ;
#80006=CARTESIAN_POINT('Ctrl Pts',(132.705912919309,-74.8258556083926,-205.3998001484)) ;
#80007=CARTESIAN_POINT('Ctrl Pts',(130.842036869422,-74.7762462333926,-205.3998001484)) ;
#80008=CARTESIAN_POINT('Ctrl Pts',(128.978160819536,-74.7266368583926,-205.3998001484)) ;
#80009=CARTESIAN_POINT('Ctrl Pts',(127.66020142537,-74.6770274833926,-204.081840754234)) ;
#80010=CARTESIAN_POINT('Ctrl Pts',(126.342242031204,-74.6274181083926,-202.763881360068)) ;
#80011=CARTESIAN_POINT('Ctrl Pts',(126.342242031204,-74.5778087333926,-200.900005310181)) ;
#80012=CARTESIAN_POINT('Ctrl Pts',(126.342242031204,-74.5281993583926,-199.036129260295)) ;
#80013=CARTESIAN_POINT('Ctrl Pts',(127.66020142537,-74.4785899833926,-197.718169866129)) ;
#80014=CARTESIAN_POINT('Ctrl Pts',(128.978160819536,-74.4289806083926,-196.400210471963)) ;
#80015=CARTESIAN_POINT('Ctrl Pts',(130.842036869422,-74.3793712333926,-196.400210471963)) ;
#80016=CARTESIAN_POINT('Ctrl Pts',(132.705912919309,-74.3297618583926,-196.400210471962)) ;
#80017=CARTESIAN_POINT('Ctrl Pts',(134.023872313475,-74.2801524833926,-197.718169866128)) ;
#80018=CARTESIAN_POINT('Ctrl Pts',(135.341831707641,-74.2305431083926,-199.036129260294)) ;
#80019=CARTESIAN_POINT('Ctrl Pts',(135.341831707641,-74.1809337333926,-200.900005310181)) ;
#80020=CARTESIAN_POINT('Ctrl Pts',(135.341831707641,-74.1313243583926,-202.763881360068)) ;
#80021=CARTESIAN_POINT('Ctrl Pts',(134.023872313475,-74.0817149833926,-204.081840754234)) ;
#80022=CARTESIAN_POINT('Ctrl Pts',(132.705912919309,-74.0321056083926,-205.3998001484)) ;
#80023=CARTESIAN_POINT('Ctrl Pts',(130.842036869422,-73.9824962333926,-205.3998001484)) ;
#80024=CARTESIAN_POINT('Ctrl Pts',(128.978160819536,-73.9328868583926,-205.3998001484)) ;
#80025=CARTESIAN_POINT('Ctrl Pts',(127.66020142537,-73.8832774833926,-204.081840754234)) ;
#80026=CARTESIAN_POINT('Ctrl Pts',(126.342242031204,-73.8336681083926,-202.763881360068)) ;
#80027=CARTESIAN_POINT('Ctrl Pts',(126.342242031204,-73.7840587333926,-200.900005310181)) ;
#80028=CARTESIAN_POINT('Ctrl Pts',(126.342242031204,-73.7344493583927,-199.036129260295)) ;
#80029=CARTESIAN_POINT('Ctrl Pts',(127.66020142537,-73.6848399833926,-197.718169866129)) ;
#80030=CARTESIAN_POINT('Ctrl Pts',(128.978160819536,-73.6352306083926,-196.400210471963)) ;
#80031=CARTESIAN_POINT('Ctrl Pts',(130.842036869422,-73.5856212333926,-196.400210471963)) ;
#80032=CARTESIAN_POINT('Ctrl Pts',(132.705912919309,-73.5360118583926,-196.400210471962)) ;
#80033=CARTESIAN_POINT('Ctrl Pts',(134.023872313475,-73.4864024833926,-197.718169866128)) ;
#80034=CARTESIAN_POINT('Ctrl Pts',(135.341831707641,-73.4367931083926,-199.036129260294)) ;
#80035=CARTESIAN_POINT('Ctrl Pts',(135.341831707641,-73.3871837333926,-200.900005310181)) ;
#80036=CARTESIAN_POINT('Ctrl Pts',(135.341831707641,-73.3375743583926,-202.763881360068)) ;
#80037=CARTESIAN_POINT('Ctrl Pts',(134.023872313475,-73.2879649833926,-204.081840754234)) ;
#80038=CARTESIAN_POINT('Ctrl Pts',(132.705912919309,-73.2383556083926,-205.3998001484)) ;
#80039=CARTESIAN_POINT('Ctrl Pts',(130.842036869422,-73.1887462333926,-205.3998001484)) ;
#80040=CARTESIAN_POINT('Ctrl Pts',(128.978160819536,-73.1391368583926,-205.3998001484)) ;
#80041=CARTESIAN_POINT('Ctrl Pts',(127.66020142537,-73.0895274833926,-204.081840754234)) ;
#80042=CARTESIAN_POINT('Ctrl Pts',(126.342242031204,-73.0399181083926,-202.763881360068)) ;
#80043=CARTESIAN_POINT('Ctrl Pts',(126.342242031204,-72.9903087333926,-200.900005310181)) ;
#80044=CARTESIAN_POINT('Ctrl Pts',(126.342242031204,-72.9406993583926,-199.036129260295)) ;
#80045=CARTESIAN_POINT('Ctrl Pts',(127.66020142537,-72.8910899833926,-197.718169866129)) ;
#80046=CARTESIAN_POINT('Ctrl Pts',(128.978160819536,-72.8414806083926,-196.400210471963)) ;
#80047=CARTESIAN_POINT('Ctrl Pts',(130.842036869422,-72.7918712333926,-196.400210471963)) ;
#80048=CARTESIAN_POINT('Ctrl Pts',(132.705912919309,-72.7422618583926,-196.400210471962)) ;
#80049=CARTESIAN_POINT('Ctrl Pts',(134.023872313475,-72.6926524833926,-197.718169866128)) ;
#80050=CARTESIAN_POINT('Ctrl Pts',(135.341831707641,-72.6430431083926,-199.036129260294)) ;
#80051=CARTESIAN_POINT('Ctrl Pts',(135.341831707641,-72.5934337333926,-200.900005310181)) ;
#80052=CARTESIAN_POINT('Ctrl Pts',(135.341831707641,-72.5438243583926,-202.763881360068)) ;
#80053=CARTESIAN_POINT('Ctrl Pts',(134.023872313475,-72.4942149833926,-204.081840754234)) ;
#80054=CARTESIAN_POINT('Ctrl Pts',(132.705912919309,-72.4446056083926,-205.3998001484)) ;
#80055=CARTESIAN_POINT('Ctrl Pts',(130.842036869422,-72.3949962333926,-205.3998001484)) ;
#80056=CARTESIAN_POINT('Ctrl Pts',(128.978160819536,-72.3453868583926,-205.3998001484)) ;
#80057=CARTESIAN_POINT('Ctrl Pts',(127.66020142537,-72.2957774833926,-204.081840754234)) ;
#80058=CARTESIAN_POINT('Ctrl Pts',(126.342242031204,-72.2461681083926,-202.763881360068)) ;
#80059=CARTESIAN_POINT('Ctrl Pts',(126.342242031204,-72.1965587333926,-200.900005310181)) ;
#80060=CARTESIAN_POINT('Ctrl Pts',(126.342242031204,-72.1469493583926,-199.036129260295)) ;
#80061=CARTESIAN_POINT('Ctrl Pts',(127.66020142537,-72.0973399833926,-197.718169866129)) ;
#80062=CARTESIAN_POINT('Ctrl Pts',(128.978160819536,-72.0477306083926,-196.400210471963)) ;
#80063=CARTESIAN_POINT('Ctrl Pts',(130.842036869422,-71.9981212333926,-196.400210471963)) ;
#80064=CARTESIAN_POINT('Ctrl Pts',(132.705912919309,-71.9485118583926,-196.400210471962)) ;
#80065=CARTESIAN_POINT('Ctrl Pts',(134.023872313475,-71.8989024833926,-197.718169866128)) ;
#80066=CARTESIAN_POINT('Ctrl Pts',(135.341831707641,-71.8492931083926,-199.036129260294)) ;
#80067=CARTESIAN_POINT('Ctrl Pts',(135.341831707641,-71.7996837333926,-200.900005310181)) ;
#80068=CARTESIAN_POINT('Ctrl Pts',(132.594636869422,-80.5295274127545,-200.900005310181)) ;
#80069=CARTESIAN_POINT('Ctrl Pts',(132.594636869422,-80.4799180377545,-201.625955999596)) ;
#80070=CARTESIAN_POINT('Ctrl Pts',(132.08131221413,-80.4303086627545,-202.139280654889)) ;
#80071=CARTESIAN_POINT('Ctrl Pts',(131.567987558838,-80.3806992877545,-202.652605310181)) ;
#80072=CARTESIAN_POINT('Ctrl Pts',(130.842036869422,-80.3310899127545,-202.652605310181)) ;
#80073=CARTESIAN_POINT('Ctrl Pts',(130.116086180007,-80.2814805377545,-202.652605310181)) ;
#80074=CARTESIAN_POINT('Ctrl Pts',(129.602761524715,-80.2318711627545,-202.139280654889)) ;
#80075=CARTESIAN_POINT('Ctrl Pts',(129.089436869422,-80.1822617877545,-201.625955999596)) ;
#80076=CARTESIAN_POINT('Ctrl Pts',(129.089436869422,-80.1326524127545,-200.900005310181)) ;
#80077=CARTESIAN_POINT('Ctrl Pts',(129.089436869422,-80.0830430377545,-200.174054620766)) ;
#80078=CARTESIAN_POINT('Ctrl Pts',(129.602761524715,-80.0334336627545,-199.660729965474)) ;
#80079=CARTESIAN_POINT('Ctrl Pts',(130.116086180007,-79.9838242877545,-199.147405310181)) ;
#80080=CARTESIAN_POINT('Ctrl Pts',(130.842036869422,-79.9342149127545,-199.147405310181)) ;
#80081=CARTESIAN_POINT('Ctrl Pts',(131.567987558837,-79.8846055377545,-199.147405310181)) ;
#80082=CARTESIAN_POINT('Ctrl Pts',(132.08131221413,-79.8349961627545,-199.660729965474)) ;
#80083=CARTESIAN_POINT('Ctrl Pts',(132.594636869422,-79.7853867877545,-200.174054620766)) ;
#80084=CARTESIAN_POINT('Ctrl Pts',(132.594636869422,-79.7357774127545,-200.900005310181)) ;
#80085=CARTESIAN_POINT('Ctrl Pts',(132.594636869422,-79.6861680377545,-201.625955999596)) ;
#80086=CARTESIAN_POINT('Ctrl Pts',(132.08131221413,-79.6365586627545,-202.139280654889)) ;
#80087=CARTESIAN_POINT('Ctrl Pts',(131.567987558838,-79.5869492877545,-202.652605310181)) ;
#80088=CARTESIAN_POINT('Ctrl Pts',(130.842036869422,-79.5373399127545,-202.652605310181)) ;
#80089=CARTESIAN_POINT('Ctrl Pts',(130.116086180007,-79.4877305377545,-202.652605310181)) ;
#80090=CARTESIAN_POINT('Ctrl Pts',(129.602761524715,-79.4381211627545,-202.139280654889)) ;
#80091=CARTESIAN_POINT('Ctrl Pts',(129.089436869422,-79.3885117877545,-201.625955999596)) ;
#80092=CARTESIAN_POINT('Ctrl Pts',(129.089436869422,-79.3389024127545,-200.900005310181)) ;
#80093=CARTESIAN_POINT('Ctrl Pts',(129.089436869422,-79.2892930377545,-200.174054620766)) ;
#80094=CARTESIAN_POINT('Ctrl Pts',(129.602761524715,-79.2396836627545,-199.660729965474)) ;
#80095=CARTESIAN_POINT('Ctrl Pts',(130.116086180007,-79.1900742877545,-199.147405310181)) ;
#80096=CARTESIAN_POINT('Ctrl Pts',(130.842036869422,-79.1404649127545,-199.147405310181)) ;
#80097=CARTESIAN_POINT('Ctrl Pts',(131.567987558837,-79.0908555377545,-199.147405310181)) ;
#80098=CARTESIAN_POINT('Ctrl Pts',(132.08131221413,-79.0412461627545,-199.660729965474)) ;
#80099=CARTESIAN_POINT('Ctrl Pts',(132.594636869422,-78.9916367877545,-200.174054620766)) ;
#80100=CARTESIAN_POINT('Ctrl Pts',(132.594636869422,-78.9420274127545,-200.900005310181)) ;
#80101=CARTESIAN_POINT('Ctrl Pts',(132.594636869422,-78.8924180377545,-201.625955999596)) ;
#80102=CARTESIAN_POINT('Ctrl Pts',(132.08131221413,-78.8428086627545,-202.139280654889)) ;
#80103=CARTESIAN_POINT('Ctrl Pts',(131.567987558838,-78.7931992877545,-202.652605310181)) ;
#80104=CARTESIAN_POINT('Ctrl Pts',(130.842036869422,-78.7435899127545,-202.652605310181)) ;
#80105=CARTESIAN_POINT('Ctrl Pts',(130.116086180007,-78.6939805377545,-202.652605310181)) ;
#80106=CARTESIAN_POINT('Ctrl Pts',(129.602761524715,-78.6443711627545,-202.139280654889)) ;
#80107=CARTESIAN_POINT('Ctrl Pts',(129.089436869422,-78.5947617877545,-201.625955999596)) ;
#80108=CARTESIAN_POINT('Ctrl Pts',(129.089436869422,-78.5451524127545,-200.900005310181)) ;
#80109=CARTESIAN_POINT('Ctrl Pts',(129.089436869422,-78.4955430377545,-200.174054620766)) ;
#80110=CARTESIAN_POINT('Ctrl Pts',(129.602761524715,-78.4459336627545,-199.660729965474)) ;
#80111=CARTESIAN_POINT('Ctrl Pts',(130.116086180007,-78.3963242877545,-199.147405310181)) ;
#80112=CARTESIAN_POINT('Ctrl Pts',(130.842036869422,-78.3467149127545,-199.147405310181)) ;
#80113=CARTESIAN_POINT('Ctrl Pts',(131.567987558837,-78.2971055377545,-199.147405310181)) ;
#80114=CARTESIAN_POINT('Ctrl Pts',(132.08131221413,-78.2474961627545,-199.660729965474)) ;
#80115=CARTESIAN_POINT('Ctrl Pts',(132.594636869422,-78.1978867877545,-200.174054620766)) ;
#80116=CARTESIAN_POINT('Ctrl Pts',(132.594636869422,-78.1482774127545,-200.900005310181)) ;
#80117=CARTESIAN_POINT('Ctrl Pts',(132.594636869422,-78.0986680377545,-201.625955999596)) ;
#80118=CARTESIAN_POINT('Ctrl Pts',(132.08131221413,-78.0490586627545,-202.139280654889)) ;
#80119=CARTESIAN_POINT('Ctrl Pts',(131.567987558838,-77.9994492877545,-202.652605310181)) ;
#80120=CARTESIAN_POINT('Ctrl Pts',(130.842036869422,-77.9498399127545,-202.652605310181)) ;
#80121=CARTESIAN_POINT('Ctrl Pts',(130.116086180007,-77.9002305377545,-202.652605310181)) ;
#80122=CARTESIAN_POINT('Ctrl Pts',(129.602761524715,-77.8506211627545,-202.139280654889)) ;
#80123=CARTESIAN_POINT('Ctrl Pts',(129.089436869422,-77.8010117877545,-201.625955999596)) ;
#80124=CARTESIAN_POINT('Ctrl Pts',(129.089436869422,-77.7514024127545,-200.900005310181)) ;
#80125=CARTESIAN_POINT('Ctrl Pts',(129.089436869422,-77.7017930377545,-200.174054620766)) ;
#80126=CARTESIAN_POINT('Ctrl Pts',(129.602761524715,-77.6521836627545,-199.660729965474)) ;
#80127=CARTESIAN_POINT('Ctrl Pts',(130.116086180007,-77.6025742877545,-199.147405310181)) ;
#80128=CARTESIAN_POINT('Ctrl Pts',(130.842036869422,-77.5529649127545,-199.147405310181)) ;
#80129=CARTESIAN_POINT('Ctrl Pts',(131.567987558837,-77.5033555377545,-199.147405310181)) ;
#80130=CARTESIAN_POINT('Ctrl Pts',(132.08131221413,-77.4537461627545,-199.660729965474)) ;
#80131=CARTESIAN_POINT('Ctrl Pts',(132.594636869422,-77.4041367877545,-200.174054620766)) ;
#80132=CARTESIAN_POINT('Ctrl Pts',(132.594636869422,-77.3545274127545,-200.900005310181)) ;
#80133=CARTESIAN_POINT('Ctrl Pts',(132.594636869422,-77.3049180377545,-201.625955999596)) ;
#80134=CARTESIAN_POINT('Ctrl Pts',(132.08131221413,-77.2553086627545,-202.139280654889)) ;
#80135=CARTESIAN_POINT('Ctrl Pts',(131.567987558838,-77.2056992877545,-202.652605310181)) ;
#80136=CARTESIAN_POINT('Ctrl Pts',(130.842036869422,-77.1560899127545,-202.652605310181)) ;
#80137=CARTESIAN_POINT('Ctrl Pts',(130.116086180007,-77.1064805377545,-202.652605310181)) ;
#80138=CARTESIAN_POINT('Ctrl Pts',(129.602761524715,-77.0568711627545,-202.139280654889)) ;
#80139=CARTESIAN_POINT('Ctrl Pts',(129.089436869422,-77.0072617877545,-201.625955999596)) ;
#80140=CARTESIAN_POINT('Ctrl Pts',(129.089436869422,-76.9576524127545,-200.900005310181)) ;
#80141=CARTESIAN_POINT('Ctrl Pts',(129.089436869422,-76.9080430377545,-200.174054620766)) ;
#80142=CARTESIAN_POINT('Ctrl Pts',(129.602761524715,-76.8584336627545,-199.660729965474)) ;
#80143=CARTESIAN_POINT('Ctrl Pts',(130.116086180007,-76.8088242877545,-199.147405310181)) ;
#80144=CARTESIAN_POINT('Ctrl Pts',(130.842036869422,-76.7592149127545,-199.147405310181)) ;
#80145=CARTESIAN_POINT('Ctrl Pts',(131.567987558837,-76.7096055377545,-199.147405310181)) ;
#80146=CARTESIAN_POINT('Ctrl Pts',(132.08131221413,-76.6599961627545,-199.660729965474)) ;
#80147=CARTESIAN_POINT('Ctrl Pts',(132.594636869422,-76.6103867877545,-200.174054620766)) ;
#80148=CARTESIAN_POINT('Ctrl Pts',(132.594636869422,-76.5607774127545,-200.900005310181)) ;
#80149=CARTESIAN_POINT('Ctrl Pts',(132.594636869422,-76.5111680377545,-201.625955999596)) ;
#80150=CARTESIAN_POINT('Ctrl Pts',(132.08131221413,-76.4615586627545,-202.139280654889)) ;
#80151=CARTESIAN_POINT('Ctrl Pts',(131.567987558838,-76.4119492877545,-202.652605310181)) ;
#80152=CARTESIAN_POINT('Ctrl Pts',(130.842036869422,-76.3623399127545,-202.652605310181)) ;
#80153=CARTESIAN_POINT('Ctrl Pts',(130.116086180007,-76.3127305377545,-202.652605310181)) ;
#80154=CARTESIAN_POINT('Ctrl Pts',(129.602761524715,-76.2631211627545,-202.139280654889)) ;
#80155=CARTESIAN_POINT('Ctrl Pts',(129.089436869422,-76.2135117877545,-201.625955999596)) ;
#80156=CARTESIAN_POINT('Ctrl Pts',(129.089436869422,-76.1639024127545,-200.900005310181)) ;
#80157=CARTESIAN_POINT('Ctrl Pts',(129.089436869422,-76.1142930377545,-200.174054620766)) ;
#80158=CARTESIAN_POINT('Ctrl Pts',(129.602761524715,-76.0646836627545,-199.660729965474)) ;
#80159=CARTESIAN_POINT('Ctrl Pts',(130.116086180007,-76.0150742877545,-199.147405310181)) ;
#80160=CARTESIAN_POINT('Ctrl Pts',(130.842036869422,-75.9654649127545,-199.147405310181)) ;
#80161=CARTESIAN_POINT('Ctrl Pts',(131.567987558837,-75.9158555377545,-199.147405310181)) ;
#80162=CARTESIAN_POINT('Ctrl Pts',(132.08131221413,-75.8662461627545,-199.660729965474)) ;
#80163=CARTESIAN_POINT('Ctrl Pts',(132.594636869422,-75.8166367877545,-200.174054620766)) ;
#80164=CARTESIAN_POINT('Ctrl Pts',(132.594636869422,-75.7670274127545,-200.900005310181)) ;
#80165=CARTESIAN_POINT('Ctrl Pts',(132.594636869422,-75.7174180377545,-201.625955999596)) ;
#80166=CARTESIAN_POINT('Ctrl Pts',(132.08131221413,-75.6678086627545,-202.139280654889)) ;
#80167=CARTESIAN_POINT('Ctrl Pts',(131.567987558837,-75.6181992877545,-202.652605310181)) ;
#80168=CARTESIAN_POINT('Ctrl Pts',(130.842036869422,-75.5685899127545,-202.652605310181)) ;
#80169=CARTESIAN_POINT('Ctrl Pts',(130.116086180007,-75.5189805377545,-202.652605310181)) ;
#80170=CARTESIAN_POINT('Ctrl Pts',(129.602761524715,-75.4693711627545,-202.139280654889)) ;
#80171=CARTESIAN_POINT('Ctrl Pts',(129.089436869422,-75.4197617877545,-201.625955999596)) ;
#80172=CARTESIAN_POINT('Ctrl Pts',(129.089436869422,-75.3701524127545,-200.900005310181)) ;
#80173=CARTESIAN_POINT('Ctrl Pts',(129.089436869422,-75.3205430377545,-200.174054620766)) ;
#80174=CARTESIAN_POINT('Ctrl Pts',(129.602761524715,-75.2709336627545,-199.660729965474)) ;
#80175=CARTESIAN_POINT('Ctrl Pts',(130.116086180007,-75.2213242877545,-199.147405310181)) ;
#80176=CARTESIAN_POINT('Ctrl Pts',(130.842036869422,-75.1717149127545,-199.147405310181)) ;
#80177=CARTESIAN_POINT('Ctrl Pts',(131.567987558837,-75.1221055377545,-199.147405310181)) ;
#80178=CARTESIAN_POINT('Ctrl Pts',(132.08131221413,-75.0724961627545,-199.660729965474)) ;
#80179=CARTESIAN_POINT('Ctrl Pts',(132.594636869422,-75.0228867877545,-200.174054620766)) ;
#80180=CARTESIAN_POINT('Ctrl Pts',(132.594636869422,-74.9732774127545,-200.900005310181)) ;
#80181=CARTESIAN_POINT('Ctrl Pts',(132.594636869422,-74.9236680377545,-201.625955999596)) ;
#80182=CARTESIAN_POINT('Ctrl Pts',(132.08131221413,-74.8740586627545,-202.139280654889)) ;
#80183=CARTESIAN_POINT('Ctrl Pts',(131.567987558837,-74.8244492877545,-202.652605310181)) ;
#80184=CARTESIAN_POINT('Ctrl Pts',(130.842036869422,-74.7748399127545,-202.652605310181)) ;
#80185=CARTESIAN_POINT('Ctrl Pts',(130.116086180007,-74.7252305377545,-202.652605310181)) ;
#80186=CARTESIAN_POINT('Ctrl Pts',(129.602761524715,-74.6756211627545,-202.139280654889)) ;
#80187=CARTESIAN_POINT('Ctrl Pts',(129.089436869422,-74.6260117877545,-201.625955999596)) ;
#80188=CARTESIAN_POINT('Ctrl Pts',(129.089436869422,-74.5764024127545,-200.900005310181)) ;
#80189=CARTESIAN_POINT('Ctrl Pts',(129.089436869422,-74.5267930377545,-200.174054620766)) ;
#80190=CARTESIAN_POINT('Ctrl Pts',(129.602761524715,-74.4771836627545,-199.660729965474)) ;
#80191=CARTESIAN_POINT('Ctrl Pts',(130.116086180007,-74.4275742877545,-199.147405310181)) ;
#80192=CARTESIAN_POINT('Ctrl Pts',(130.842036869422,-74.3779649127545,-199.147405310181)) ;
#80193=CARTESIAN_POINT('Ctrl Pts',(131.567987558837,-74.3283555377545,-199.147405310181)) ;
#80194=CARTESIAN_POINT('Ctrl Pts',(132.08131221413,-74.2787461627545,-199.660729965474)) ;
#80195=CARTESIAN_POINT('Ctrl Pts',(132.594636869422,-74.2291367877545,-200.174054620766)) ;
#80196=CARTESIAN_POINT('Ctrl Pts',(132.594636869422,-74.1795274127545,-200.900005310181)) ;
#80197=CARTESIAN_POINT('Ctrl Pts',(132.594636869422,-74.1299180377545,-201.625955999596)) ;
#80198=CARTESIAN_POINT('Ctrl Pts',(132.08131221413,-74.0803086627545,-202.139280654889)) ;
#80199=CARTESIAN_POINT('Ctrl Pts',(131.567987558837,-74.0306992877545,-202.652605310181)) ;
#80200=CARTESIAN_POINT('Ctrl Pts',(130.842036869422,-73.9810899127545,-202.652605310181)) ;
#80201=CARTESIAN_POINT('Ctrl Pts',(130.116086180007,-73.9314805377545,-202.652605310181)) ;
#80202=CARTESIAN_POINT('Ctrl Pts',(129.602761524715,-73.8818711627545,-202.139280654889)) ;
#80203=CARTESIAN_POINT('Ctrl Pts',(129.089436869422,-73.8322617877545,-201.625955999596)) ;
#80204=CARTESIAN_POINT('Ctrl Pts',(129.089436869422,-73.7826524127545,-200.900005310181)) ;
#80205=CARTESIAN_POINT('Ctrl Pts',(129.089436869422,-73.7330430377545,-200.174054620766)) ;
#80206=CARTESIAN_POINT('Ctrl Pts',(129.602761524715,-73.6834336627545,-199.660729965474)) ;
#80207=CARTESIAN_POINT('Ctrl Pts',(130.116086180007,-73.6338242877545,-199.147405310181)) ;
#80208=CARTESIAN_POINT('Ctrl Pts',(130.842036869422,-73.5842149127545,-199.147405310181)) ;
#80209=CARTESIAN_POINT('Ctrl Pts',(131.567987558837,-73.5346055377545,-199.147405310181)) ;
#80210=CARTESIAN_POINT('Ctrl Pts',(132.08131221413,-73.4849961627545,-199.660729965474)) ;
#80211=CARTESIAN_POINT('Ctrl Pts',(132.594636869422,-73.4353867877545,-200.174054620766)) ;
#80212=CARTESIAN_POINT('Ctrl Pts',(132.594636869422,-73.3857774127545,-200.900005310181)) ;
#80213=CARTESIAN_POINT('Ctrl Pts',(132.079081121232,-80.8271836627545,-200.900005310181)) ;
#80214=CARTESIAN_POINT('Ctrl Pts',(132.079081121232,-80.7775742877545,-201.412405816536)) ;
#80215=CARTESIAN_POINT('Ctrl Pts',(131.716759248505,-80.7279649127545,-201.774727689263)) ;
#80216=CARTESIAN_POINT('Ctrl Pts',(131.354437375778,-80.6783555377545,-202.137049561991)) ;
#80217=CARTESIAN_POINT('Ctrl Pts',(130.842036869422,-80.6287461627545,-202.137049561991)) ;
#80218=CARTESIAN_POINT('Ctrl Pts',(130.329636363067,-80.5791367877545,-202.137049561991)) ;
#80219=CARTESIAN_POINT('Ctrl Pts',(129.96731449034,-80.5295274127545,-201.774727689264)) ;
#80220=CARTESIAN_POINT('Ctrl Pts',(129.604992617613,-80.4799180377545,-201.412405816536)) ;
#80221=CARTESIAN_POINT('Ctrl Pts',(129.604992617613,-80.4303086627545,-200.900005310181)) ;
#80222=CARTESIAN_POINT('Ctrl Pts',(129.604992617613,-80.3806992877545,-200.387604803826)) ;
#80223=CARTESIAN_POINT('Ctrl Pts',(129.96731449034,-80.3310899127545,-200.025282931099)) ;
#80224=CARTESIAN_POINT('Ctrl Pts',(130.329636363067,-80.2814805377545,-199.662961058372)) ;
#80225=CARTESIAN_POINT('Ctrl Pts',(130.842036869422,-80.2318711627545,-199.662961058372)) ;
#80226=CARTESIAN_POINT('Ctrl Pts',(131.354437375778,-80.1822617877545,-199.662961058371)) ;
#80227=CARTESIAN_POINT('Ctrl Pts',(131.716759248505,-80.1326524127545,-200.025282931099)) ;
#80228=CARTESIAN_POINT('Ctrl Pts',(132.079081121232,-80.0830430377545,-200.387604803826)) ;
#80229=CARTESIAN_POINT('Ctrl Pts',(132.079081121232,-80.0334336627545,-200.900005310181)) ;
#80230=CARTESIAN_POINT('Ctrl Pts',(132.079081121232,-79.9838242877545,-201.412405816536)) ;
#80231=CARTESIAN_POINT('Ctrl Pts',(131.716759248505,-79.9342149127545,-201.774727689263)) ;
#80232=CARTESIAN_POINT('Ctrl Pts',(131.354437375778,-79.8846055377545,-202.137049561991)) ;
#80233=CARTESIAN_POINT('Ctrl Pts',(130.842036869422,-79.8349961627545,-202.137049561991)) ;
#80234=CARTESIAN_POINT('Ctrl Pts',(130.329636363067,-79.7853867877545,-202.137049561991)) ;
#80235=CARTESIAN_POINT('Ctrl Pts',(129.96731449034,-79.7357774127545,-201.774727689264)) ;
#80236=CARTESIAN_POINT('Ctrl Pts',(129.604992617613,-79.6861680377545,-201.412405816536)) ;
#80237=CARTESIAN_POINT('Ctrl Pts',(129.604992617613,-79.6365586627545,-200.900005310181)) ;
#80238=CARTESIAN_POINT('Ctrl Pts',(129.604992617613,-79.5869492877545,-200.387604803826)) ;
#80239=CARTESIAN_POINT('Ctrl Pts',(129.96731449034,-79.5373399127545,-200.025282931099)) ;
#80240=CARTESIAN_POINT('Ctrl Pts',(130.329636363067,-79.4877305377545,-199.662961058372)) ;
#80241=CARTESIAN_POINT('Ctrl Pts',(130.842036869422,-79.4381211627545,-199.662961058372)) ;
#80242=CARTESIAN_POINT('Ctrl Pts',(131.354437375778,-79.3885117877545,-199.662961058371)) ;
#80243=CARTESIAN_POINT('Ctrl Pts',(131.716759248505,-79.3389024127545,-200.025282931099)) ;
#80244=CARTESIAN_POINT('Ctrl Pts',(132.079081121232,-79.2892930377545,-200.387604803826)) ;
#80245=CARTESIAN_POINT('Ctrl Pts',(132.079081121232,-79.2396836627545,-200.900005310181)) ;
#80246=CARTESIAN_POINT('Ctrl Pts',(132.079081121232,-79.1900742877545,-201.412405816536)) ;
#80247=CARTESIAN_POINT('Ctrl Pts',(131.716759248505,-79.1404649127545,-201.774727689263)) ;
#80248=CARTESIAN_POINT('Ctrl Pts',(131.354437375778,-79.0908555377545,-202.137049561991)) ;
#80249=CARTESIAN_POINT('Ctrl Pts',(130.842036869422,-79.0412461627545,-202.137049561991)) ;
#80250=CARTESIAN_POINT('Ctrl Pts',(130.329636363067,-78.9916367877545,-202.137049561991)) ;
#80251=CARTESIAN_POINT('Ctrl Pts',(129.96731449034,-78.9420274127545,-201.774727689264)) ;
#80252=CARTESIAN_POINT('Ctrl Pts',(129.604992617613,-78.8924180377545,-201.412405816536)) ;
#80253=CARTESIAN_POINT('Ctrl Pts',(129.604992617613,-78.8428086627545,-200.900005310181)) ;
#80254=CARTESIAN_POINT('Ctrl Pts',(129.604992617613,-78.7931992877545,-200.387604803826)) ;
#80255=CARTESIAN_POINT('Ctrl Pts',(129.96731449034,-78.7435899127545,-200.025282931099)) ;
#80256=CARTESIAN_POINT('Ctrl Pts',(130.329636363067,-78.6939805377545,-199.662961058372)) ;
#80257=CARTESIAN_POINT('Ctrl Pts',(130.842036869422,-78.6443711627545,-199.662961058372)) ;
#80258=CARTESIAN_POINT('Ctrl Pts',(131.354437375778,-78.5947617877545,-199.662961058371)) ;
#80259=CARTESIAN_POINT('Ctrl Pts',(131.716759248505,-78.5451524127545,-200.025282931099)) ;
#80260=CARTESIAN_POINT('Ctrl Pts',(132.079081121232,-78.4955430377545,-200.387604803826)) ;
#80261=CARTESIAN_POINT('Ctrl Pts',(132.079081121232,-78.4459336627545,-200.900005310181)) ;
#80262=CARTESIAN_POINT('Ctrl Pts',(132.079081121232,-78.3963242877545,-201.412405816536)) ;
#80263=CARTESIAN_POINT('Ctrl Pts',(131.716759248505,-78.3467149127545,-201.774727689263)) ;
#80264=CARTESIAN_POINT('Ctrl Pts',(131.354437375778,-78.2971055377545,-202.137049561991)) ;
#80265=CARTESIAN_POINT('Ctrl Pts',(130.842036869422,-78.2474961627545,-202.137049561991)) ;
#80266=CARTESIAN_POINT('Ctrl Pts',(130.329636363067,-78.1978867877545,-202.137049561991)) ;
#80267=CARTESIAN_POINT('Ctrl Pts',(129.96731449034,-78.1482774127545,-201.774727689264)) ;
#80268=CARTESIAN_POINT('Ctrl Pts',(129.604992617613,-78.0986680377545,-201.412405816536)) ;
#80269=CARTESIAN_POINT('Ctrl Pts',(129.604992617613,-78.0490586627545,-200.900005310181)) ;
#80270=CARTESIAN_POINT('Ctrl Pts',(129.604992617613,-77.9994492877545,-200.387604803826)) ;
#80271=CARTESIAN_POINT('Ctrl Pts',(129.96731449034,-77.9498399127545,-200.025282931099)) ;
#80272=CARTESIAN_POINT('Ctrl Pts',(130.329636363067,-77.9002305377545,-199.662961058372)) ;
#80273=CARTESIAN_POINT('Ctrl Pts',(130.842036869422,-77.8506211627545,-199.662961058372)) ;
#80274=CARTESIAN_POINT('Ctrl Pts',(131.354437375778,-77.8010117877545,-199.662961058371)) ;
#80275=CARTESIAN_POINT('Ctrl Pts',(131.716759248505,-77.7514024127545,-200.025282931099)) ;
#80276=CARTESIAN_POINT('Ctrl Pts',(132.079081121232,-77.7017930377545,-200.387604803826)) ;
#80277=CARTESIAN_POINT('Ctrl Pts',(132.079081121232,-77.6521836627545,-200.900005310181)) ;
#80278=CARTESIAN_POINT('Ctrl Pts',(132.079081121232,-77.6025742877545,-201.412405816536)) ;
#80279=CARTESIAN_POINT('Ctrl Pts',(131.716759248505,-77.5529649127545,-201.774727689263)) ;
#80280=CARTESIAN_POINT('Ctrl Pts',(131.354437375778,-77.5033555377545,-202.137049561991)) ;
#80281=CARTESIAN_POINT('Ctrl Pts',(130.842036869422,-77.4537461627545,-202.137049561991)) ;
#80282=CARTESIAN_POINT('Ctrl Pts',(130.329636363067,-77.4041367877545,-202.137049561991)) ;
#80283=CARTESIAN_POINT('Ctrl Pts',(129.96731449034,-77.3545274127545,-201.774727689264)) ;
#80284=CARTESIAN_POINT('Ctrl Pts',(129.604992617613,-77.3049180377545,-201.412405816536)) ;
#80285=CARTESIAN_POINT('Ctrl Pts',(129.604992617613,-77.2553086627545,-200.900005310181)) ;
#80286=CARTESIAN_POINT('Ctrl Pts',(129.604992617613,-77.2056992877545,-200.387604803826)) ;
#80287=CARTESIAN_POINT('Ctrl Pts',(129.96731449034,-77.1560899127545,-200.025282931099)) ;
#80288=CARTESIAN_POINT('Ctrl Pts',(130.329636363067,-77.1064805377545,-199.662961058372)) ;
#80289=CARTESIAN_POINT('Ctrl Pts',(130.842036869422,-77.0568711627545,-199.662961058372)) ;
#80290=CARTESIAN_POINT('Ctrl Pts',(131.354437375778,-77.0072617877545,-199.662961058371)) ;
#80291=CARTESIAN_POINT('Ctrl Pts',(131.716759248505,-76.9576524127545,-200.025282931099)) ;
#80292=CARTESIAN_POINT('Ctrl Pts',(132.079081121232,-76.9080430377545,-200.387604803826)) ;
#80293=CARTESIAN_POINT('Ctrl Pts',(132.079081121232,-76.8584336627545,-200.900005310181)) ;
#80294=CARTESIAN_POINT('Ctrl Pts',(132.079081121232,-76.8088242877545,-201.412405816536)) ;
#80295=CARTESIAN_POINT('Ctrl Pts',(131.716759248505,-76.7592149127545,-201.774727689263)) ;
#80296=CARTESIAN_POINT('Ctrl Pts',(131.354437375778,-76.7096055377545,-202.137049561991)) ;
#80297=CARTESIAN_POINT('Ctrl Pts',(130.842036869422,-76.6599961627545,-202.137049561991)) ;
#80298=CARTESIAN_POINT('Ctrl Pts',(130.329636363067,-76.6103867877545,-202.137049561991)) ;
#80299=CARTESIAN_POINT('Ctrl Pts',(129.96731449034,-76.5607774127545,-201.774727689264)) ;
#80300=CARTESIAN_POINT('Ctrl Pts',(129.604992617613,-76.5111680377545,-201.412405816536)) ;
#80301=CARTESIAN_POINT('Ctrl Pts',(129.604992617613,-76.4615586627545,-200.900005310181)) ;
#80302=CARTESIAN_POINT('Ctrl Pts',(129.604992617613,-76.4119492877545,-200.387604803826)) ;
#80303=CARTESIAN_POINT('Ctrl Pts',(129.96731449034,-76.3623399127545,-200.025282931099)) ;
#80304=CARTESIAN_POINT('Ctrl Pts',(130.329636363067,-76.3127305377545,-199.662961058372)) ;
#80305=CARTESIAN_POINT('Ctrl Pts',(130.842036869422,-76.2631211627545,-199.662961058372)) ;
#80306=CARTESIAN_POINT('Ctrl Pts',(131.354437375778,-76.2135117877545,-199.662961058371)) ;
#80307=CARTESIAN_POINT('Ctrl Pts',(131.716759248505,-76.1639024127545,-200.025282931099)) ;
#80308=CARTESIAN_POINT('Ctrl Pts',(132.079081121232,-76.1142930377545,-200.387604803826)) ;
#80309=CARTESIAN_POINT('Ctrl Pts',(132.079081121232,-76.0646836627545,-200.900005310181)) ;
#80310=CARTESIAN_POINT('Ctrl Pts',(132.079081121232,-76.0150742877545,-201.412405816536)) ;
#80311=CARTESIAN_POINT('Ctrl Pts',(131.716759248505,-75.9654649127545,-201.774727689263)) ;
#80312=CARTESIAN_POINT('Ctrl Pts',(131.354437375778,-75.9158555377545,-202.137049561991)) ;
#80313=CARTESIAN_POINT('Ctrl Pts',(130.842036869422,-75.8662461627545,-202.137049561991)) ;
#80314=CARTESIAN_POINT('Ctrl Pts',(130.329636363067,-75.8166367877545,-202.137049561991)) ;
#80315=CARTESIAN_POINT('Ctrl Pts',(129.96731449034,-75.7670274127545,-201.774727689264)) ;
#80316=CARTESIAN_POINT('Ctrl Pts',(129.604992617613,-75.7174180377545,-201.412405816536)) ;
#80317=CARTESIAN_POINT('Ctrl Pts',(129.604992617613,-75.6678086627545,-200.900005310181)) ;
#80318=CARTESIAN_POINT('Ctrl Pts',(129.604992617613,-75.6181992877545,-200.387604803826)) ;
#80319=CARTESIAN_POINT('Ctrl Pts',(129.96731449034,-75.5685899127545,-200.025282931099)) ;
#80320=CARTESIAN_POINT('Ctrl Pts',(130.329636363067,-75.5189805377545,-199.662961058372)) ;
#80321=CARTESIAN_POINT('Ctrl Pts',(130.842036869422,-75.4693711627545,-199.662961058372)) ;
#80322=CARTESIAN_POINT('Ctrl Pts',(131.354437375778,-75.4197617877545,-199.662961058371)) ;
#80323=CARTESIAN_POINT('Ctrl Pts',(131.716759248505,-75.3701524127545,-200.025282931099)) ;
#80324=CARTESIAN_POINT('Ctrl Pts',(132.079081121232,-75.3205430377545,-200.387604803826)) ;
#80325=CARTESIAN_POINT('Ctrl Pts',(132.079081121232,-75.2709336627545,-200.900005310181)) ;
#80326=CARTESIAN_POINT('Ctrl Pts',(132.079081121232,-75.2213242877545,-201.412405816536)) ;
#80327=CARTESIAN_POINT('Ctrl Pts',(131.716759248505,-75.1717149127545,-201.774727689263)) ;
#80328=CARTESIAN_POINT('Ctrl Pts',(131.354437375778,-75.1221055377545,-202.137049561991)) ;
#80329=CARTESIAN_POINT('Ctrl Pts',(130.842036869422,-75.0724961627545,-202.137049561991)) ;
#80330=CARTESIAN_POINT('Ctrl Pts',(130.329636363067,-75.0228867877545,-202.137049561991)) ;
#80331=CARTESIAN_POINT('Ctrl Pts',(129.96731449034,-74.9732774127545,-201.774727689264)) ;
#80332=CARTESIAN_POINT('Ctrl Pts',(129.604992617613,-74.9236680377545,-201.412405816536)) ;
#80333=CARTESIAN_POINT('Ctrl Pts',(129.604992617613,-74.8740586627545,-200.900005310181)) ;
#80334=CARTESIAN_POINT('Ctrl Pts',(129.604992617613,-74.8244492877545,-200.387604803826)) ;
#80335=CARTESIAN_POINT('Ctrl Pts',(129.96731449034,-74.7748399127545,-200.025282931099)) ;
#80336=CARTESIAN_POINT('Ctrl Pts',(130.329636363067,-74.7252305377545,-199.662961058372)) ;
#80337=CARTESIAN_POINT('Ctrl Pts',(130.842036869422,-74.6756211627545,-199.662961058372)) ;
#80338=CARTESIAN_POINT('Ctrl Pts',(131.354437375778,-74.6260117877545,-199.662961058371)) ;
#80339=CARTESIAN_POINT('Ctrl Pts',(131.716759248505,-74.5764024127545,-200.025282931099)) ;
#80340=CARTESIAN_POINT('Ctrl Pts',(132.079081121232,-74.5267930377545,-200.387604803826)) ;
#80341=CARTESIAN_POINT('Ctrl Pts',(132.079081121232,-74.4771836627545,-200.900005310181)) ;
#80342=CARTESIAN_POINT('Ctrl Pts',(132.079081121232,-74.4275742877545,-201.412405816536)) ;
#80343=CARTESIAN_POINT('Ctrl Pts',(131.716759248505,-74.3779649127545,-201.774727689263)) ;
#80344=CARTESIAN_POINT('Ctrl Pts',(131.354437375778,-74.3283555377545,-202.137049561991)) ;
#80345=CARTESIAN_POINT('Ctrl Pts',(130.842036869422,-74.2787461627545,-202.137049561991)) ;
#80346=CARTESIAN_POINT('Ctrl Pts',(130.329636363067,-74.2291367877545,-202.137049561991)) ;
#80347=CARTESIAN_POINT('Ctrl Pts',(129.96731449034,-74.1795274127545,-201.774727689264)) ;
#80348=CARTESIAN_POINT('Ctrl Pts',(129.604992617613,-74.1299180377545,-201.412405816536)) ;
#80349=CARTESIAN_POINT('Ctrl Pts',(129.604992617613,-74.0803086627545,-200.900005310181)) ;
#80350=CARTESIAN_POINT('Ctrl Pts',(129.604992617613,-74.0306992877545,-200.387604803826)) ;
#80351=CARTESIAN_POINT('Ctrl Pts',(129.96731449034,-73.9810899127545,-200.025282931099)) ;
#80352=CARTESIAN_POINT('Ctrl Pts',(130.329636363067,-73.9314805377545,-199.662961058372)) ;
#80353=CARTESIAN_POINT('Ctrl Pts',(130.842036869422,-73.8818711627545,-199.662961058372)) ;
#80354=CARTESIAN_POINT('Ctrl Pts',(131.354437375778,-73.8322617877545,-199.662961058371)) ;
#80355=CARTESIAN_POINT('Ctrl Pts',(131.716759248505,-73.7826524127545,-200.025282931099)) ;
#80356=CARTESIAN_POINT('Ctrl Pts',(132.079081121232,-73.7330430377545,-200.387604803826)) ;
#80357=CARTESIAN_POINT('Ctrl Pts',(132.079081121232,-73.6834336627545,-200.900005310181)) ;
#80358=CARTESIAN_POINT('Ctrl Pts',(131.259739170827,-81.3002309583791,-200.900005310181)) ;
#80359=CARTESIAN_POINT('Ctrl Pts',(131.259739170827,-81.2506215833791,-201.073023268457)) ;
#80360=CARTESIAN_POINT('Ctrl Pts',(131.137396999263,-81.2010122083791,-201.195365440022)) ;
#80361=CARTESIAN_POINT('Ctrl Pts',(131.015054827699,-81.1514028333791,-201.317707611586)) ;
#80362=CARTESIAN_POINT('Ctrl Pts',(130.842036869422,-81.1017934583791,-201.317707611586)) ;
#80363=CARTESIAN_POINT('Ctrl Pts',(130.669018911146,-81.0521840833791,-201.317707611586)) ;
#80364=CARTESIAN_POINT('Ctrl Pts',(130.546676739582,-81.0025747083791,-201.195365440022)) ;
#80365=CARTESIAN_POINT('Ctrl Pts',(130.424334568018,-80.9529653333791,-201.073023268457)) ;
#80366=CARTESIAN_POINT('Ctrl Pts',(130.424334568018,-80.9033559583791,-200.900005310181)) ;
#80367=CARTESIAN_POINT('Ctrl Pts',(130.424334568018,-80.8537465833791,-200.726987351905)) ;
#80368=CARTESIAN_POINT('Ctrl Pts',(130.546676739582,-80.8041372083791,-200.604645180341)) ;
#80369=CARTESIAN_POINT('Ctrl Pts',(130.669018911146,-80.7545278333791,-200.482303008776)) ;
#80370=CARTESIAN_POINT('Ctrl Pts',(130.842036869422,-80.7049184583791,-200.482303008776)) ;
#80371=CARTESIAN_POINT('Ctrl Pts',(131.015054827699,-80.6553090833791,-200.482303008776)) ;
#80372=CARTESIAN_POINT('Ctrl Pts',(131.137396999263,-80.6056997083791,-200.604645180341)) ;
#80373=CARTESIAN_POINT('Ctrl Pts',(131.259739170827,-80.5560903333791,-200.726987351905)) ;
#80374=CARTESIAN_POINT('Ctrl Pts',(131.259739170827,-80.5064809583791,-200.900005310181)) ;
#80375=CARTESIAN_POINT('Ctrl Pts',(131.259739170827,-80.4568715833791,-201.073023268457)) ;
#80376=CARTESIAN_POINT('Ctrl Pts',(131.137396999263,-80.4072622083791,-201.195365440022)) ;
#80377=CARTESIAN_POINT('Ctrl Pts',(131.015054827699,-80.3576528333791,-201.317707611586)) ;
#80378=CARTESIAN_POINT('Ctrl Pts',(130.842036869422,-80.3080434583791,-201.317707611586)) ;
#80379=CARTESIAN_POINT('Ctrl Pts',(130.669018911146,-80.2584340833791,-201.317707611586)) ;
#80380=CARTESIAN_POINT('Ctrl Pts',(130.546676739582,-80.2088247083791,-201.195365440022)) ;
#80381=CARTESIAN_POINT('Ctrl Pts',(130.424334568018,-80.1592153333791,-201.073023268457)) ;
#80382=CARTESIAN_POINT('Ctrl Pts',(130.424334568018,-80.1096059583791,-200.900005310181)) ;
#80383=CARTESIAN_POINT('Ctrl Pts',(130.424334568018,-80.0599965833791,-200.726987351905)) ;
#80384=CARTESIAN_POINT('Ctrl Pts',(130.546676739582,-80.0103872083791,-200.604645180341)) ;
#80385=CARTESIAN_POINT('Ctrl Pts',(130.669018911146,-79.9607778333791,-200.482303008776)) ;
#80386=CARTESIAN_POINT('Ctrl Pts',(130.842036869422,-79.9111684583791,-200.482303008776)) ;
#80387=CARTESIAN_POINT('Ctrl Pts',(131.015054827699,-79.8615590833791,-200.482303008776)) ;
#80388=CARTESIAN_POINT('Ctrl Pts',(131.137396999263,-79.8119497083791,-200.604645180341)) ;
#80389=CARTESIAN_POINT('Ctrl Pts',(131.259739170827,-79.7623403333791,-200.726987351905)) ;
#80390=CARTESIAN_POINT('Ctrl Pts',(131.259739170827,-79.7127309583791,-200.900005310181)) ;
#80391=CARTESIAN_POINT('Ctrl Pts',(131.259739170827,-79.6631215833791,-201.073023268457)) ;
#80392=CARTESIAN_POINT('Ctrl Pts',(131.137396999263,-79.6135122083791,-201.195365440022)) ;
#80393=CARTESIAN_POINT('Ctrl Pts',(131.015054827699,-79.5639028333791,-201.317707611586)) ;
#80394=CARTESIAN_POINT('Ctrl Pts',(130.842036869422,-79.5142934583791,-201.317707611586)) ;
#80395=CARTESIAN_POINT('Ctrl Pts',(130.669018911146,-79.4646840833791,-201.317707611586)) ;
#80396=CARTESIAN_POINT('Ctrl Pts',(130.546676739582,-79.4150747083791,-201.195365440022)) ;
#80397=CARTESIAN_POINT('Ctrl Pts',(130.424334568018,-79.3654653333791,-201.073023268457)) ;
#80398=CARTESIAN_POINT('Ctrl Pts',(130.424334568018,-79.3158559583791,-200.900005310181)) ;
#80399=CARTESIAN_POINT('Ctrl Pts',(130.424334568018,-79.2662465833791,-200.726987351905)) ;
#80400=CARTESIAN_POINT('Ctrl Pts',(130.546676739582,-79.2166372083791,-200.604645180341)) ;
#80401=CARTESIAN_POINT('Ctrl Pts',(130.669018911146,-79.1670278333791,-200.482303008776)) ;
#80402=CARTESIAN_POINT('Ctrl Pts',(130.842036869422,-79.1174184583791,-200.482303008776)) ;
#80403=CARTESIAN_POINT('Ctrl Pts',(131.015054827699,-79.0678090833791,-200.482303008776)) ;
#80404=CARTESIAN_POINT('Ctrl Pts',(131.137396999263,-79.0181997083791,-200.604645180341)) ;
#80405=CARTESIAN_POINT('Ctrl Pts',(131.259739170827,-78.9685903333791,-200.726987351905)) ;
#80406=CARTESIAN_POINT('Ctrl Pts',(131.259739170827,-78.9189809583791,-200.900005310181)) ;
#80407=CARTESIAN_POINT('Ctrl Pts',(131.259739170827,-78.8693715833791,-201.073023268457)) ;
#80408=CARTESIAN_POINT('Ctrl Pts',(131.137396999263,-78.8197622083791,-201.195365440022)) ;
#80409=CARTESIAN_POINT('Ctrl Pts',(131.015054827699,-78.7701528333791,-201.317707611586)) ;
#80410=CARTESIAN_POINT('Ctrl Pts',(130.842036869422,-78.7205434583791,-201.317707611586)) ;
#80411=CARTESIAN_POINT('Ctrl Pts',(130.669018911146,-78.6709340833791,-201.317707611586)) ;
#80412=CARTESIAN_POINT('Ctrl Pts',(130.546676739582,-78.6213247083791,-201.195365440022)) ;
#80413=CARTESIAN_POINT('Ctrl Pts',(130.424334568018,-78.5717153333791,-201.073023268457)) ;
#80414=CARTESIAN_POINT('Ctrl Pts',(130.424334568018,-78.5221059583791,-200.900005310181)) ;
#80415=CARTESIAN_POINT('Ctrl Pts',(130.424334568018,-78.4724965833791,-200.726987351905)) ;
#80416=CARTESIAN_POINT('Ctrl Pts',(130.546676739582,-78.4228872083791,-200.604645180341)) ;
#80417=CARTESIAN_POINT('Ctrl Pts',(130.669018911146,-78.3732778333791,-200.482303008776)) ;
#80418=CARTESIAN_POINT('Ctrl Pts',(130.842036869422,-78.3236684583791,-200.482303008776)) ;
#80419=CARTESIAN_POINT('Ctrl Pts',(131.015054827699,-78.2740590833791,-200.482303008776)) ;
#80420=CARTESIAN_POINT('Ctrl Pts',(131.137396999263,-78.2244497083791,-200.604645180341)) ;
#80421=CARTESIAN_POINT('Ctrl Pts',(131.259739170827,-78.1748403333791,-200.726987351905)) ;
#80422=CARTESIAN_POINT('Ctrl Pts',(131.259739170827,-78.1252309583791,-200.900005310181)) ;
#80423=CARTESIAN_POINT('Ctrl Pts',(131.259739170827,-78.0756215833791,-201.073023268457)) ;
#80424=CARTESIAN_POINT('Ctrl Pts',(131.137396999263,-78.0260122083791,-201.195365440022)) ;
#80425=CARTESIAN_POINT('Ctrl Pts',(131.015054827699,-77.9764028333791,-201.317707611586)) ;
#80426=CARTESIAN_POINT('Ctrl Pts',(130.842036869422,-77.9267934583791,-201.317707611586)) ;
#80427=CARTESIAN_POINT('Ctrl Pts',(130.669018911146,-77.8771840833791,-201.317707611586)) ;
#80428=CARTESIAN_POINT('Ctrl Pts',(130.546676739582,-77.8275747083791,-201.195365440022)) ;
#80429=CARTESIAN_POINT('Ctrl Pts',(130.424334568018,-77.7779653333791,-201.073023268457)) ;
#80430=CARTESIAN_POINT('Ctrl Pts',(130.424334568018,-77.7283559583791,-200.900005310181)) ;
#80431=CARTESIAN_POINT('Ctrl Pts',(130.424334568018,-77.6787465833791,-200.726987351905)) ;
#80432=CARTESIAN_POINT('Ctrl Pts',(130.546676739582,-77.6291372083791,-200.604645180341)) ;
#80433=CARTESIAN_POINT('Ctrl Pts',(130.669018911146,-77.5795278333791,-200.482303008776)) ;
#80434=CARTESIAN_POINT('Ctrl Pts',(130.842036869422,-77.5299184583791,-200.482303008776)) ;
#80435=CARTESIAN_POINT('Ctrl Pts',(131.015054827699,-77.4803090833791,-200.482303008776)) ;
#80436=CARTESIAN_POINT('Ctrl Pts',(131.137396999263,-77.4306997083791,-200.604645180341)) ;
#80437=CARTESIAN_POINT('Ctrl Pts',(131.259739170827,-77.3810903333791,-200.726987351905)) ;
#80438=CARTESIAN_POINT('Ctrl Pts',(131.259739170827,-77.3314809583791,-200.900005310181)) ;
#80439=CARTESIAN_POINT('Ctrl Pts',(131.259739170827,-77.2818715833791,-201.073023268457)) ;
#80440=CARTESIAN_POINT('Ctrl Pts',(131.137396999263,-77.2322622083791,-201.195365440022)) ;
#80441=CARTESIAN_POINT('Ctrl Pts',(131.015054827699,-77.1826528333791,-201.317707611586)) ;
#80442=CARTESIAN_POINT('Ctrl Pts',(130.842036869422,-77.1330434583791,-201.317707611586)) ;
#80443=CARTESIAN_POINT('Ctrl Pts',(130.669018911146,-77.0834340833791,-201.317707611586)) ;
#80444=CARTESIAN_POINT('Ctrl Pts',(130.546676739582,-77.0338247083791,-201.195365440022)) ;
#80445=CARTESIAN_POINT('Ctrl Pts',(130.424334568018,-76.9842153333791,-201.073023268457)) ;
#80446=CARTESIAN_POINT('Ctrl Pts',(130.424334568018,-76.9346059583791,-200.900005310181)) ;
#80447=CARTESIAN_POINT('Ctrl Pts',(130.424334568018,-76.8849965833791,-200.726987351905)) ;
#80448=CARTESIAN_POINT('Ctrl Pts',(130.546676739582,-76.8353872083791,-200.604645180341)) ;
#80449=CARTESIAN_POINT('Ctrl Pts',(130.669018911146,-76.7857778333791,-200.482303008776)) ;
#80450=CARTESIAN_POINT('Ctrl Pts',(130.842036869422,-76.7361684583791,-200.482303008776)) ;
#80451=CARTESIAN_POINT('Ctrl Pts',(131.015054827699,-76.6865590833791,-200.482303008776)) ;
#80452=CARTESIAN_POINT('Ctrl Pts',(131.137396999263,-76.6369497083791,-200.604645180341)) ;
#80453=CARTESIAN_POINT('Ctrl Pts',(131.259739170827,-76.5873403333791,-200.726987351905)) ;
#80454=CARTESIAN_POINT('Ctrl Pts',(131.259739170827,-76.5377309583791,-200.900005310181)) ;
#80455=CARTESIAN_POINT('Ctrl Pts',(131.259739170827,-76.4881215833791,-201.073023268457)) ;
#80456=CARTESIAN_POINT('Ctrl Pts',(131.137396999263,-76.4385122083791,-201.195365440022)) ;
#80457=CARTESIAN_POINT('Ctrl Pts',(131.015054827699,-76.3889028333791,-201.317707611586)) ;
#80458=CARTESIAN_POINT('Ctrl Pts',(130.842036869422,-76.3392934583791,-201.317707611586)) ;
#80459=CARTESIAN_POINT('Ctrl Pts',(130.669018911146,-76.2896840833791,-201.317707611586)) ;
#80460=CARTESIAN_POINT('Ctrl Pts',(130.546676739582,-76.2400747083791,-201.195365440022)) ;
#80461=CARTESIAN_POINT('Ctrl Pts',(130.424334568018,-76.1904653333791,-201.073023268457)) ;
#80462=CARTESIAN_POINT('Ctrl Pts',(130.424334568018,-76.1408559583791,-200.900005310181)) ;
#80463=CARTESIAN_POINT('Ctrl Pts',(130.424334568018,-76.0912465833791,-200.726987351905)) ;
#80464=CARTESIAN_POINT('Ctrl Pts',(130.546676739582,-76.0416372083791,-200.604645180341)) ;
#80465=CARTESIAN_POINT('Ctrl Pts',(130.669018911146,-75.9920278333791,-200.482303008776)) ;
#80466=CARTESIAN_POINT('Ctrl Pts',(130.842036869422,-75.9424184583791,-200.482303008776)) ;
#80467=CARTESIAN_POINT('Ctrl Pts',(131.015054827699,-75.8928090833791,-200.482303008776)) ;
#80468=CARTESIAN_POINT('Ctrl Pts',(131.137396999263,-75.8431997083791,-200.604645180341)) ;
#80469=CARTESIAN_POINT('Ctrl Pts',(131.259739170827,-75.7935903333791,-200.726987351905)) ;
#80470=CARTESIAN_POINT('Ctrl Pts',(131.259739170827,-75.7439809583791,-200.900005310181)) ;
#80471=CARTESIAN_POINT('Ctrl Pts',(131.259739170827,-75.6943715833791,-201.073023268457)) ;
#80472=CARTESIAN_POINT('Ctrl Pts',(131.137396999263,-75.6447622083791,-201.195365440022)) ;
#80473=CARTESIAN_POINT('Ctrl Pts',(131.015054827699,-75.5951528333791,-201.317707611586)) ;
#80474=CARTESIAN_POINT('Ctrl Pts',(130.842036869422,-75.5455434583791,-201.317707611586)) ;
#80475=CARTESIAN_POINT('Ctrl Pts',(130.669018911146,-75.4959340833791,-201.317707611586)) ;
#80476=CARTESIAN_POINT('Ctrl Pts',(130.546676739582,-75.4463247083791,-201.195365440022)) ;
#80477=CARTESIAN_POINT('Ctrl Pts',(130.424334568018,-75.3967153333791,-201.073023268457)) ;
#80478=CARTESIAN_POINT('Ctrl Pts',(130.424334568018,-75.3471059583791,-200.900005310181)) ;
#80479=CARTESIAN_POINT('Ctrl Pts',(130.424334568018,-75.2974965833791,-200.726987351905)) ;
#80480=CARTESIAN_POINT('Ctrl Pts',(130.546676739582,-75.2478872083791,-200.604645180341)) ;
#80481=CARTESIAN_POINT('Ctrl Pts',(130.669018911146,-75.1982778333791,-200.482303008776)) ;
#80482=CARTESIAN_POINT('Ctrl Pts',(130.842036869422,-75.1486684583791,-200.482303008776)) ;
#80483=CARTESIAN_POINT('Ctrl Pts',(131.015054827699,-75.0990590833791,-200.482303008776)) ;
#80484=CARTESIAN_POINT('Ctrl Pts',(131.137396999263,-75.0494497083791,-200.604645180341)) ;
#80485=CARTESIAN_POINT('Ctrl Pts',(131.259739170827,-74.9998403333791,-200.726987351905)) ;
#80486=CARTESIAN_POINT('Ctrl Pts',(131.259739170827,-74.9502309583791,-200.900005310181)) ;
#80487=CARTESIAN_POINT('Ctrl Pts',(131.259739170827,-74.9006215833791,-201.073023268457)) ;
#80488=CARTESIAN_POINT('Ctrl Pts',(131.137396999263,-74.8510122083791,-201.195365440022)) ;
#80489=CARTESIAN_POINT('Ctrl Pts',(131.015054827699,-74.8014028333791,-201.317707611586)) ;
#80490=CARTESIAN_POINT('Ctrl Pts',(130.842036869422,-74.7517934583791,-201.317707611586)) ;
#80491=CARTESIAN_POINT('Ctrl Pts',(130.669018911146,-74.7021840833791,-201.317707611586)) ;
#80492=CARTESIAN_POINT('Ctrl Pts',(130.546676739582,-74.6525747083791,-201.195365440022)) ;
#80493=CARTESIAN_POINT('Ctrl Pts',(130.424334568018,-74.6029653333791,-201.073023268457)) ;
#80494=CARTESIAN_POINT('Ctrl Pts',(130.424334568018,-74.5533559583791,-200.900005310181)) ;
#80495=CARTESIAN_POINT('Ctrl Pts',(130.424334568018,-74.5037465833791,-200.726987351905)) ;
#80496=CARTESIAN_POINT('Ctrl Pts',(130.546676739582,-74.4541372083791,-200.604645180341)) ;
#80497=CARTESIAN_POINT('Ctrl Pts',(130.669018911146,-74.4045278333791,-200.482303008776)) ;
#80498=CARTESIAN_POINT('Ctrl Pts',(130.842036869422,-74.3549184583791,-200.482303008776)) ;
#80499=CARTESIAN_POINT('Ctrl Pts',(131.015054827699,-74.3053090833791,-200.482303008776)) ;
#80500=CARTESIAN_POINT('Ctrl Pts',(131.137396999263,-74.2556997083791,-200.604645180341)) ;
#80501=CARTESIAN_POINT('Ctrl Pts',(131.259739170827,-74.2060903333791,-200.726987351905)) ;
#80502=CARTESIAN_POINT('Ctrl Pts',(131.259739170827,-74.1564809583791,-200.900005310181)) ;
#80503=CARTESIAN_POINT('Ctrl Pts',(132.079081121232,-80.9264024127545,-200.900005310181)) ;
#80504=CARTESIAN_POINT('Ctrl Pts',(132.079081121232,-80.8767930377545,-201.412405816536)) ;
#80505=CARTESIAN_POINT('Ctrl Pts',(131.716759248505,-80.8271836627545,-201.774727689263)) ;
#80506=CARTESIAN_POINT('Ctrl Pts',(131.354437375778,-80.7775742877545,-202.137049561991)) ;
#80507=CARTESIAN_POINT('Ctrl Pts',(130.842036869422,-80.7279649127545,-202.137049561991)) ;
#80508=CARTESIAN_POINT('Ctrl Pts',(130.329636363067,-80.6783555377545,-202.137049561991)) ;
#80509=CARTESIAN_POINT('Ctrl Pts',(129.96731449034,-80.6287461627545,-201.774727689264)) ;
#80510=CARTESIAN_POINT('Ctrl Pts',(129.604992617613,-80.5791367877545,-201.412405816536)) ;
#80511=CARTESIAN_POINT('Ctrl Pts',(129.604992617613,-80.5295274127545,-200.900005310181)) ;
#80512=CARTESIAN_POINT('Ctrl Pts',(129.604992617613,-80.4799180377545,-200.387604803826)) ;
#80513=CARTESIAN_POINT('Ctrl Pts',(129.96731449034,-80.4303086627545,-200.025282931099)) ;
#80514=CARTESIAN_POINT('Ctrl Pts',(130.329636363067,-80.3806992877545,-199.662961058372)) ;
#80515=CARTESIAN_POINT('Ctrl Pts',(130.842036869422,-80.3310899127545,-199.662961058372)) ;
#80516=CARTESIAN_POINT('Ctrl Pts',(131.354437375778,-80.2814805377545,-199.662961058371)) ;
#80517=CARTESIAN_POINT('Ctrl Pts',(131.716759248505,-80.2318711627545,-200.025282931099)) ;
#80518=CARTESIAN_POINT('Ctrl Pts',(132.079081121232,-80.1822617877545,-200.387604803826)) ;
#80519=CARTESIAN_POINT('Ctrl Pts',(132.079081121232,-80.1326524127545,-200.900005310181)) ;
#80520=CARTESIAN_POINT('Ctrl Pts',(132.079081121232,-80.0830430377545,-201.412405816536)) ;
#80521=CARTESIAN_POINT('Ctrl Pts',(131.716759248505,-80.0334336627545,-201.774727689263)) ;
#80522=CARTESIAN_POINT('Ctrl Pts',(131.354437375778,-79.9838242877545,-202.137049561991)) ;
#80523=CARTESIAN_POINT('Ctrl Pts',(130.842036869422,-79.9342149127545,-202.137049561991)) ;
#80524=CARTESIAN_POINT('Ctrl Pts',(130.329636363067,-79.8846055377545,-202.137049561991)) ;
#80525=CARTESIAN_POINT('Ctrl Pts',(129.96731449034,-79.8349961627545,-201.774727689264)) ;
#80526=CARTESIAN_POINT('Ctrl Pts',(129.604992617613,-79.7853867877545,-201.412405816536)) ;
#80527=CARTESIAN_POINT('Ctrl Pts',(129.604992617613,-79.7357774127545,-200.900005310181)) ;
#80528=CARTESIAN_POINT('Ctrl Pts',(129.604992617613,-79.6861680377545,-200.387604803826)) ;
#80529=CARTESIAN_POINT('Ctrl Pts',(129.96731449034,-79.6365586627545,-200.025282931099)) ;
#80530=CARTESIAN_POINT('Ctrl Pts',(130.329636363067,-79.5869492877545,-199.662961058372)) ;
#80531=CARTESIAN_POINT('Ctrl Pts',(130.842036869422,-79.5373399127545,-199.662961058372)) ;
#80532=CARTESIAN_POINT('Ctrl Pts',(131.354437375778,-79.4877305377545,-199.662961058371)) ;
#80533=CARTESIAN_POINT('Ctrl Pts',(131.716759248505,-79.4381211627545,-200.025282931099)) ;
#80534=CARTESIAN_POINT('Ctrl Pts',(132.079081121232,-79.3885117877545,-200.387604803826)) ;
#80535=CARTESIAN_POINT('Ctrl Pts',(132.079081121232,-79.3389024127545,-200.900005310181)) ;
#80536=CARTESIAN_POINT('Ctrl Pts',(132.079081121232,-79.2892930377545,-201.412405816536)) ;
#80537=CARTESIAN_POINT('Ctrl Pts',(131.716759248505,-79.2396836627545,-201.774727689263)) ;
#80538=CARTESIAN_POINT('Ctrl Pts',(131.354437375778,-79.1900742877545,-202.137049561991)) ;
#80539=CARTESIAN_POINT('Ctrl Pts',(130.842036869422,-79.1404649127545,-202.137049561991)) ;
#80540=CARTESIAN_POINT('Ctrl Pts',(130.329636363067,-79.0908555377545,-202.137049561991)) ;
#80541=CARTESIAN_POINT('Ctrl Pts',(129.96731449034,-79.0412461627545,-201.774727689264)) ;
#80542=CARTESIAN_POINT('Ctrl Pts',(129.604992617613,-78.9916367877545,-201.412405816536)) ;
#80543=CARTESIAN_POINT('Ctrl Pts',(129.604992617613,-78.9420274127545,-200.900005310181)) ;
#80544=CARTESIAN_POINT('Ctrl Pts',(129.604992617613,-78.8924180377545,-200.387604803826)) ;
#80545=CARTESIAN_POINT('Ctrl Pts',(129.96731449034,-78.8428086627545,-200.025282931099)) ;
#80546=CARTESIAN_POINT('Ctrl Pts',(130.329636363067,-78.7931992877545,-199.662961058372)) ;
#80547=CARTESIAN_POINT('Ctrl Pts',(130.842036869422,-78.7435899127545,-199.662961058372)) ;
#80548=CARTESIAN_POINT('Ctrl Pts',(131.354437375778,-78.6939805377545,-199.662961058371)) ;
#80549=CARTESIAN_POINT('Ctrl Pts',(131.716759248505,-78.6443711627545,-200.025282931099)) ;
#80550=CARTESIAN_POINT('Ctrl Pts',(132.079081121232,-78.5947617877545,-200.387604803826)) ;
#80551=CARTESIAN_POINT('Ctrl Pts',(132.079081121232,-78.5451524127545,-200.900005310181)) ;
#80552=CARTESIAN_POINT('Ctrl Pts',(132.079081121232,-78.4955430377545,-201.412405816536)) ;
#80553=CARTESIAN_POINT('Ctrl Pts',(131.716759248505,-78.4459336627545,-201.774727689263)) ;
#80554=CARTESIAN_POINT('Ctrl Pts',(131.354437375778,-78.3963242877545,-202.137049561991)) ;
#80555=CARTESIAN_POINT('Ctrl Pts',(130.842036869422,-78.3467149127545,-202.137049561991)) ;
#80556=CARTESIAN_POINT('Ctrl Pts',(130.329636363067,-78.2971055377545,-202.137049561991)) ;
#80557=CARTESIAN_POINT('Ctrl Pts',(129.96731449034,-78.2474961627545,-201.774727689264)) ;
#80558=CARTESIAN_POINT('Ctrl Pts',(129.604992617613,-78.1978867877545,-201.412405816536)) ;
#80559=CARTESIAN_POINT('Ctrl Pts',(129.604992617613,-78.1482774127545,-200.900005310181)) ;
#80560=CARTESIAN_POINT('Ctrl Pts',(129.604992617613,-78.0986680377545,-200.387604803826)) ;
#80561=CARTESIAN_POINT('Ctrl Pts',(129.96731449034,-78.0490586627545,-200.025282931099)) ;
#80562=CARTESIAN_POINT('Ctrl Pts',(130.329636363067,-77.9994492877545,-199.662961058372)) ;
#80563=CARTESIAN_POINT('Ctrl Pts',(130.842036869422,-77.9498399127545,-199.662961058372)) ;
#80564=CARTESIAN_POINT('Ctrl Pts',(131.354437375778,-77.9002305377545,-199.662961058371)) ;
#80565=CARTESIAN_POINT('Ctrl Pts',(131.716759248505,-77.8506211627545,-200.025282931099)) ;
#80566=CARTESIAN_POINT('Ctrl Pts',(132.079081121232,-77.8010117877545,-200.387604803826)) ;
#80567=CARTESIAN_POINT('Ctrl Pts',(132.079081121232,-77.7514024127545,-200.900005310181)) ;
#80568=CARTESIAN_POINT('Ctrl Pts',(132.079081121232,-77.7017930377545,-201.412405816536)) ;
#80569=CARTESIAN_POINT('Ctrl Pts',(131.716759248505,-77.6521836627545,-201.774727689263)) ;
#80570=CARTESIAN_POINT('Ctrl Pts',(131.354437375778,-77.6025742877545,-202.137049561991)) ;
#80571=CARTESIAN_POINT('Ctrl Pts',(130.842036869422,-77.5529649127545,-202.137049561991)) ;
#80572=CARTESIAN_POINT('Ctrl Pts',(130.329636363067,-77.5033555377545,-202.137049561991)) ;
#80573=CARTESIAN_POINT('Ctrl Pts',(129.96731449034,-77.4537461627545,-201.774727689264)) ;
#80574=CARTESIAN_POINT('Ctrl Pts',(129.604992617613,-77.4041367877545,-201.412405816536)) ;
#80575=CARTESIAN_POINT('Ctrl Pts',(129.604992617613,-77.3545274127545,-200.900005310181)) ;
#80576=CARTESIAN_POINT('Ctrl Pts',(129.604992617613,-77.3049180377545,-200.387604803826)) ;
#80577=CARTESIAN_POINT('Ctrl Pts',(129.96731449034,-77.2553086627545,-200.025282931099)) ;
#80578=CARTESIAN_POINT('Ctrl Pts',(130.329636363067,-77.2056992877545,-199.662961058372)) ;
#80579=CARTESIAN_POINT('Ctrl Pts',(130.842036869422,-77.1560899127545,-199.662961058372)) ;
#80580=CARTESIAN_POINT('Ctrl Pts',(131.354437375778,-77.1064805377545,-199.662961058371)) ;
#80581=CARTESIAN_POINT('Ctrl Pts',(131.716759248505,-77.0568711627545,-200.025282931099)) ;
#80582=CARTESIAN_POINT('Ctrl Pts',(132.079081121232,-77.0072617877545,-200.387604803826)) ;
#80583=CARTESIAN_POINT('Ctrl Pts',(132.079081121232,-76.9576524127545,-200.900005310181)) ;
#80584=CARTESIAN_POINT('Ctrl Pts',(132.079081121232,-76.9080430377545,-201.412405816536)) ;
#80585=CARTESIAN_POINT('Ctrl Pts',(131.716759248505,-76.8584336627545,-201.774727689263)) ;
#80586=CARTESIAN_POINT('Ctrl Pts',(131.354437375778,-76.8088242877545,-202.137049561991)) ;
#80587=CARTESIAN_POINT('Ctrl Pts',(130.842036869422,-76.7592149127545,-202.137049561991)) ;
#80588=CARTESIAN_POINT('Ctrl Pts',(130.329636363067,-76.7096055377545,-202.137049561991)) ;
#80589=CARTESIAN_POINT('Ctrl Pts',(129.96731449034,-76.6599961627545,-201.774727689264)) ;
#80590=CARTESIAN_POINT('Ctrl Pts',(129.604992617613,-76.6103867877545,-201.412405816536)) ;
#80591=CARTESIAN_POINT('Ctrl Pts',(129.604992617613,-76.5607774127545,-200.900005310181)) ;
#80592=CARTESIAN_POINT('Ctrl Pts',(129.604992617613,-76.5111680377545,-200.387604803826)) ;
#80593=CARTESIAN_POINT('Ctrl Pts',(129.96731449034,-76.4615586627545,-200.025282931099)) ;
#80594=CARTESIAN_POINT('Ctrl Pts',(130.329636363067,-76.4119492877545,-199.662961058372)) ;
#80595=CARTESIAN_POINT('Ctrl Pts',(130.842036869422,-76.3623399127545,-199.662961058372)) ;
#80596=CARTESIAN_POINT('Ctrl Pts',(131.354437375778,-76.3127305377545,-199.662961058371)) ;
#80597=CARTESIAN_POINT('Ctrl Pts',(131.716759248505,-76.2631211627545,-200.025282931099)) ;
#80598=CARTESIAN_POINT('Ctrl Pts',(132.079081121232,-76.2135117877545,-200.387604803826)) ;
#80599=CARTESIAN_POINT('Ctrl Pts',(132.079081121232,-76.1639024127545,-200.900005310181)) ;
#80600=CARTESIAN_POINT('Ctrl Pts',(132.079081121232,-76.1142930377545,-201.412405816536)) ;
#80601=CARTESIAN_POINT('Ctrl Pts',(131.716759248505,-76.0646836627545,-201.774727689263)) ;
#80602=CARTESIAN_POINT('Ctrl Pts',(131.354437375778,-76.0150742877545,-202.137049561991)) ;
#80603=CARTESIAN_POINT('Ctrl Pts',(130.842036869422,-75.9654649127545,-202.137049561991)) ;
#80604=CARTESIAN_POINT('Ctrl Pts',(130.329636363067,-75.9158555377545,-202.137049561991)) ;
#80605=CARTESIAN_POINT('Ctrl Pts',(129.96731449034,-75.8662461627545,-201.774727689264)) ;
#80606=CARTESIAN_POINT('Ctrl Pts',(129.604992617613,-75.8166367877545,-201.412405816536)) ;
#80607=CARTESIAN_POINT('Ctrl Pts',(129.604992617613,-75.7670274127545,-200.900005310181)) ;
#80608=CARTESIAN_POINT('Ctrl Pts',(129.604992617613,-75.7174180377545,-200.387604803826)) ;
#80609=CARTESIAN_POINT('Ctrl Pts',(129.96731449034,-75.6678086627545,-200.025282931099)) ;
#80610=CARTESIAN_POINT('Ctrl Pts',(130.329636363067,-75.6181992877545,-199.662961058372)) ;
#80611=CARTESIAN_POINT('Ctrl Pts',(130.842036869422,-75.5685899127545,-199.662961058372)) ;
#80612=CARTESIAN_POINT('Ctrl Pts',(131.354437375778,-75.5189805377545,-199.662961058371)) ;
#80613=CARTESIAN_POINT('Ctrl Pts',(131.716759248505,-75.4693711627545,-200.025282931099)) ;
#80614=CARTESIAN_POINT('Ctrl Pts',(132.079081121232,-75.4197617877545,-200.387604803826)) ;
#80615=CARTESIAN_POINT('Ctrl Pts',(132.079081121232,-75.3701524127545,-200.900005310181)) ;
#80616=CARTESIAN_POINT('Ctrl Pts',(132.079081121232,-75.3205430377545,-201.412405816536)) ;
#80617=CARTESIAN_POINT('Ctrl Pts',(131.716759248505,-75.2709336627545,-201.774727689263)) ;
#80618=CARTESIAN_POINT('Ctrl Pts',(131.354437375778,-75.2213242877545,-202.137049561991)) ;
#80619=CARTESIAN_POINT('Ctrl Pts',(130.842036869422,-75.1717149127545,-202.137049561991)) ;
#80620=CARTESIAN_POINT('Ctrl Pts',(130.329636363067,-75.1221055377545,-202.137049561991)) ;
#80621=CARTESIAN_POINT('Ctrl Pts',(129.96731449034,-75.0724961627545,-201.774727689264)) ;
#80622=CARTESIAN_POINT('Ctrl Pts',(129.604992617613,-75.0228867877545,-201.412405816536)) ;
#80623=CARTESIAN_POINT('Ctrl Pts',(129.604992617613,-74.9732774127545,-200.900005310181)) ;
#80624=CARTESIAN_POINT('Ctrl Pts',(129.604992617613,-74.9236680377545,-200.387604803826)) ;
#80625=CARTESIAN_POINT('Ctrl Pts',(129.96731449034,-74.8740586627545,-200.025282931099)) ;
#80626=CARTESIAN_POINT('Ctrl Pts',(130.329636363067,-74.8244492877545,-199.662961058372)) ;
#80627=CARTESIAN_POINT('Ctrl Pts',(130.842036869422,-74.7748399127545,-199.662961058372)) ;
#80628=CARTESIAN_POINT('Ctrl Pts',(131.354437375778,-74.7252305377545,-199.662961058371)) ;
#80629=CARTESIAN_POINT('Ctrl Pts',(131.716759248505,-74.6756211627545,-200.025282931099)) ;
#80630=CARTESIAN_POINT('Ctrl Pts',(132.079081121232,-74.6260117877545,-200.387604803826)) ;
#80631=CARTESIAN_POINT('Ctrl Pts',(132.079081121232,-74.5764024127545,-200.900005310181)) ;
#80632=CARTESIAN_POINT('Ctrl Pts',(132.079081121232,-74.5267930377545,-201.412405816536)) ;
#80633=CARTESIAN_POINT('Ctrl Pts',(131.716759248505,-74.4771836627545,-201.774727689263)) ;
#80634=CARTESIAN_POINT('Ctrl Pts',(131.354437375778,-74.4275742877545,-202.137049561991)) ;
#80635=CARTESIAN_POINT('Ctrl Pts',(130.842036869422,-74.3779649127545,-202.137049561991)) ;
#80636=CARTESIAN_POINT('Ctrl Pts',(130.329636363067,-74.3283555377545,-202.137049561991)) ;
#80637=CARTESIAN_POINT('Ctrl Pts',(129.96731449034,-74.2787461627545,-201.774727689264)) ;
#80638=CARTESIAN_POINT('Ctrl Pts',(129.604992617613,-74.2291367877545,-201.412405816536)) ;
#80639=CARTESIAN_POINT('Ctrl Pts',(129.604992617613,-74.1795274127545,-200.900005310181)) ;
#80640=CARTESIAN_POINT('Ctrl Pts',(129.604992617613,-74.1299180377545,-200.387604803826)) ;
#80641=CARTESIAN_POINT('Ctrl Pts',(129.96731449034,-74.0803086627545,-200.025282931099)) ;
#80642=CARTESIAN_POINT('Ctrl Pts',(130.329636363067,-74.0306992877545,-199.662961058372)) ;
#80643=CARTESIAN_POINT('Ctrl Pts',(130.842036869422,-73.9810899127545,-199.662961058372)) ;
#80644=CARTESIAN_POINT('Ctrl Pts',(131.354437375778,-73.9314805377545,-199.662961058371)) ;
#80645=CARTESIAN_POINT('Ctrl Pts',(131.716759248505,-73.8818711627545,-200.025282931099)) ;
#80646=CARTESIAN_POINT('Ctrl Pts',(132.079081121232,-73.8322617877545,-200.387604803826)) ;
#80647=CARTESIAN_POINT('Ctrl Pts',(132.079081121232,-73.7826524127545,-200.900005310181)) ;
#80648=CARTESIAN_POINT('Ctrl Pts',(132.594659680647,-81.224071832821,-200.900005310181)) ;
#80649=CARTESIAN_POINT('Ctrl Pts',(132.594659680647,-81.174462457821,-201.625965448315)) ;
#80650=CARTESIAN_POINT('Ctrl Pts',(132.081328344101,-81.124853082821,-202.13929678486)) ;
#80651=CARTESIAN_POINT('Ctrl Pts',(131.567997007556,-81.075243707821,-202.652628121405)) ;
#80652=CARTESIAN_POINT('Ctrl Pts',(130.842036869422,-81.025634332821,-202.652628121405)) ;
#80653=CARTESIAN_POINT('Ctrl Pts',(130.116076731289,-80.976024957821,-202.652628121405)) ;
#80654=CARTESIAN_POINT('Ctrl Pts',(129.602745394743,-80.926415582821,-202.13929678486)) ;
#80655=CARTESIAN_POINT('Ctrl Pts',(129.089414058198,-80.876806207821,-201.625965448315)) ;
#80656=CARTESIAN_POINT('Ctrl Pts',(129.089414058198,-80.827196832821,-200.900005310181)) ;
#80657=CARTESIAN_POINT('Ctrl Pts',(129.089414058198,-80.777587457821,-200.174045172048)) ;
#80658=CARTESIAN_POINT('Ctrl Pts',(129.602745394743,-80.727978082821,-199.660713835502)) ;
#80659=CARTESIAN_POINT('Ctrl Pts',(130.116076731289,-80.678368707821,-199.147382498957)) ;
#80660=CARTESIAN_POINT('Ctrl Pts',(130.842036869422,-80.628759332821,-199.147382498957)) ;
#80661=CARTESIAN_POINT('Ctrl Pts',(131.567997007556,-80.579149957821,-199.147382498957)) ;
#80662=CARTESIAN_POINT('Ctrl Pts',(132.081328344101,-80.529540582821,-199.660713835502)) ;
#80663=CARTESIAN_POINT('Ctrl Pts',(132.594659680647,-80.479931207821,-200.174045172047)) ;
#80664=CARTESIAN_POINT('Ctrl Pts',(132.594659680647,-80.430321832821,-200.900005310181)) ;
#80665=CARTESIAN_POINT('Ctrl Pts',(132.594659680647,-80.380712457821,-201.625965448315)) ;
#80666=CARTESIAN_POINT('Ctrl Pts',(132.081328344101,-80.331103082821,-202.13929678486)) ;
#80667=CARTESIAN_POINT('Ctrl Pts',(131.567997007556,-80.281493707821,-202.652628121405)) ;
#80668=CARTESIAN_POINT('Ctrl Pts',(130.842036869422,-80.231884332821,-202.652628121405)) ;
#80669=CARTESIAN_POINT('Ctrl Pts',(130.116076731289,-80.182274957821,-202.652628121405)) ;
#80670=CARTESIAN_POINT('Ctrl Pts',(129.602745394743,-80.132665582821,-202.13929678486)) ;
#80671=CARTESIAN_POINT('Ctrl Pts',(129.089414058198,-80.083056207821,-201.625965448315)) ;
#80672=CARTESIAN_POINT('Ctrl Pts',(129.089414058198,-80.033446832821,-200.900005310181)) ;
#80673=CARTESIAN_POINT('Ctrl Pts',(129.089414058198,-79.983837457821,-200.174045172048)) ;
#80674=CARTESIAN_POINT('Ctrl Pts',(129.602745394743,-79.934228082821,-199.660713835502)) ;
#80675=CARTESIAN_POINT('Ctrl Pts',(130.116076731289,-79.884618707821,-199.147382498957)) ;
#80676=CARTESIAN_POINT('Ctrl Pts',(130.842036869422,-79.835009332821,-199.147382498957)) ;
#80677=CARTESIAN_POINT('Ctrl Pts',(131.567997007556,-79.785399957821,-199.147382498957)) ;
#80678=CARTESIAN_POINT('Ctrl Pts',(132.081328344101,-79.735790582821,-199.660713835502)) ;
#80679=CARTESIAN_POINT('Ctrl Pts',(132.594659680647,-79.686181207821,-200.174045172047)) ;
#80680=CARTESIAN_POINT('Ctrl Pts',(132.594659680647,-79.636571832821,-200.900005310181)) ;
#80681=CARTESIAN_POINT('Ctrl Pts',(132.594659680647,-79.586962457821,-201.625965448315)) ;
#80682=CARTESIAN_POINT('Ctrl Pts',(132.081328344101,-79.537353082821,-202.13929678486)) ;
#80683=CARTESIAN_POINT('Ctrl Pts',(131.567997007556,-79.487743707821,-202.652628121405)) ;
#80684=CARTESIAN_POINT('Ctrl Pts',(130.842036869422,-79.438134332821,-202.652628121405)) ;
#80685=CARTESIAN_POINT('Ctrl Pts',(130.116076731289,-79.388524957821,-202.652628121405)) ;
#80686=CARTESIAN_POINT('Ctrl Pts',(129.602745394743,-79.338915582821,-202.13929678486)) ;
#80687=CARTESIAN_POINT('Ctrl Pts',(129.089414058198,-79.289306207821,-201.625965448315)) ;
#80688=CARTESIAN_POINT('Ctrl Pts',(129.089414058198,-79.239696832821,-200.900005310181)) ;
#80689=CARTESIAN_POINT('Ctrl Pts',(129.089414058198,-79.190087457821,-200.174045172048)) ;
#80690=CARTESIAN_POINT('Ctrl Pts',(129.602745394743,-79.140478082821,-199.660713835502)) ;
#80691=CARTESIAN_POINT('Ctrl Pts',(130.116076731289,-79.090868707821,-199.147382498957)) ;
#80692=CARTESIAN_POINT('Ctrl Pts',(130.842036869422,-79.041259332821,-199.147382498957)) ;
#80693=CARTESIAN_POINT('Ctrl Pts',(131.567997007556,-78.991649957821,-199.147382498957)) ;
#80694=CARTESIAN_POINT('Ctrl Pts',(132.081328344101,-78.942040582821,-199.660713835502)) ;
#80695=CARTESIAN_POINT('Ctrl Pts',(132.594659680647,-78.892431207821,-200.174045172047)) ;
#80696=CARTESIAN_POINT('Ctrl Pts',(132.594659680647,-78.842821832821,-200.900005310181)) ;
#80697=CARTESIAN_POINT('Ctrl Pts',(132.594659680647,-78.793212457821,-201.625965448315)) ;
#80698=CARTESIAN_POINT('Ctrl Pts',(132.081328344101,-78.743603082821,-202.13929678486)) ;
#80699=CARTESIAN_POINT('Ctrl Pts',(131.567997007556,-78.693993707821,-202.652628121405)) ;
#80700=CARTESIAN_POINT('Ctrl Pts',(130.842036869422,-78.644384332821,-202.652628121405)) ;
#80701=CARTESIAN_POINT('Ctrl Pts',(130.116076731289,-78.594774957821,-202.652628121405)) ;
#80702=CARTESIAN_POINT('Ctrl Pts',(129.602745394743,-78.545165582821,-202.13929678486)) ;
#80703=CARTESIAN_POINT('Ctrl Pts',(129.089414058198,-78.495556207821,-201.625965448315)) ;
#80704=CARTESIAN_POINT('Ctrl Pts',(129.089414058198,-78.445946832821,-200.900005310181)) ;
#80705=CARTESIAN_POINT('Ctrl Pts',(129.089414058198,-78.396337457821,-200.174045172048)) ;
#80706=CARTESIAN_POINT('Ctrl Pts',(129.602745394743,-78.346728082821,-199.660713835502)) ;
#80707=CARTESIAN_POINT('Ctrl Pts',(130.116076731289,-78.297118707821,-199.147382498957)) ;
#80708=CARTESIAN_POINT('Ctrl Pts',(130.842036869422,-78.247509332821,-199.147382498957)) ;
#80709=CARTESIAN_POINT('Ctrl Pts',(131.567997007556,-78.197899957821,-199.147382498957)) ;
#80710=CARTESIAN_POINT('Ctrl Pts',(132.081328344101,-78.148290582821,-199.660713835502)) ;
#80711=CARTESIAN_POINT('Ctrl Pts',(132.594659680647,-78.098681207821,-200.174045172047)) ;
#80712=CARTESIAN_POINT('Ctrl Pts',(132.594659680647,-78.049071832821,-200.900005310181)) ;
#80713=CARTESIAN_POINT('Ctrl Pts',(132.594659680647,-77.999462457821,-201.625965448315)) ;
#80714=CARTESIAN_POINT('Ctrl Pts',(132.081328344101,-77.949853082821,-202.13929678486)) ;
#80715=CARTESIAN_POINT('Ctrl Pts',(131.567997007556,-77.900243707821,-202.652628121405)) ;
#80716=CARTESIAN_POINT('Ctrl Pts',(130.842036869422,-77.850634332821,-202.652628121405)) ;
#80717=CARTESIAN_POINT('Ctrl Pts',(130.116076731289,-77.801024957821,-202.652628121405)) ;
#80718=CARTESIAN_POINT('Ctrl Pts',(129.602745394743,-77.751415582821,-202.13929678486)) ;
#80719=CARTESIAN_POINT('Ctrl Pts',(129.089414058198,-77.701806207821,-201.625965448315)) ;
#80720=CARTESIAN_POINT('Ctrl Pts',(129.089414058198,-77.652196832821,-200.900005310181)) ;
#80721=CARTESIAN_POINT('Ctrl Pts',(129.089414058198,-77.602587457821,-200.174045172048)) ;
#80722=CARTESIAN_POINT('Ctrl Pts',(129.602745394743,-77.552978082821,-199.660713835502)) ;
#80723=CARTESIAN_POINT('Ctrl Pts',(130.116076731289,-77.503368707821,-199.147382498957)) ;
#80724=CARTESIAN_POINT('Ctrl Pts',(130.842036869422,-77.453759332821,-199.147382498957)) ;
#80725=CARTESIAN_POINT('Ctrl Pts',(131.567997007556,-77.404149957821,-199.147382498957)) ;
#80726=CARTESIAN_POINT('Ctrl Pts',(132.081328344101,-77.354540582821,-199.660713835502)) ;
#80727=CARTESIAN_POINT('Ctrl Pts',(132.594659680647,-77.304931207821,-200.174045172047)) ;
#80728=CARTESIAN_POINT('Ctrl Pts',(132.594659680647,-77.255321832821,-200.900005310181)) ;
#80729=CARTESIAN_POINT('Ctrl Pts',(132.594659680647,-77.205712457821,-201.625965448315)) ;
#80730=CARTESIAN_POINT('Ctrl Pts',(132.081328344101,-77.156103082821,-202.13929678486)) ;
#80731=CARTESIAN_POINT('Ctrl Pts',(131.567997007556,-77.106493707821,-202.652628121405)) ;
#80732=CARTESIAN_POINT('Ctrl Pts',(130.842036869422,-77.056884332821,-202.652628121405)) ;
#80733=CARTESIAN_POINT('Ctrl Pts',(130.116076731289,-77.007274957821,-202.652628121405)) ;
#80734=CARTESIAN_POINT('Ctrl Pts',(129.602745394743,-76.957665582821,-202.13929678486)) ;
#80735=CARTESIAN_POINT('Ctrl Pts',(129.089414058198,-76.908056207821,-201.625965448315)) ;
#80736=CARTESIAN_POINT('Ctrl Pts',(129.089414058198,-76.858446832821,-200.900005310181)) ;
#80737=CARTESIAN_POINT('Ctrl Pts',(129.089414058198,-76.808837457821,-200.174045172048)) ;
#80738=CARTESIAN_POINT('Ctrl Pts',(129.602745394743,-76.759228082821,-199.660713835502)) ;
#80739=CARTESIAN_POINT('Ctrl Pts',(130.116076731289,-76.709618707821,-199.147382498957)) ;
#80740=CARTESIAN_POINT('Ctrl Pts',(130.842036869422,-76.660009332821,-199.147382498957)) ;
#80741=CARTESIAN_POINT('Ctrl Pts',(131.567997007556,-76.610399957821,-199.147382498957)) ;
#80742=CARTESIAN_POINT('Ctrl Pts',(132.081328344101,-76.560790582821,-199.660713835502)) ;
#80743=CARTESIAN_POINT('Ctrl Pts',(132.594659680647,-76.511181207821,-200.174045172047)) ;
#80744=CARTESIAN_POINT('Ctrl Pts',(132.594659680647,-76.461571832821,-200.900005310181)) ;
#80745=CARTESIAN_POINT('Ctrl Pts',(132.594659680647,-76.411962457821,-201.625965448315)) ;
#80746=CARTESIAN_POINT('Ctrl Pts',(132.081328344101,-76.362353082821,-202.13929678486)) ;
#80747=CARTESIAN_POINT('Ctrl Pts',(131.567997007556,-76.312743707821,-202.652628121405)) ;
#80748=CARTESIAN_POINT('Ctrl Pts',(130.842036869422,-76.263134332821,-202.652628121405)) ;
#80749=CARTESIAN_POINT('Ctrl Pts',(130.116076731289,-76.213524957821,-202.652628121405)) ;
#80750=CARTESIAN_POINT('Ctrl Pts',(129.602745394743,-76.163915582821,-202.13929678486)) ;
#80751=CARTESIAN_POINT('Ctrl Pts',(129.089414058198,-76.114306207821,-201.625965448315)) ;
#80752=CARTESIAN_POINT('Ctrl Pts',(129.089414058198,-76.064696832821,-200.900005310181)) ;
#80753=CARTESIAN_POINT('Ctrl Pts',(129.089414058198,-76.015087457821,-200.174045172048)) ;
#80754=CARTESIAN_POINT('Ctrl Pts',(129.602745394743,-75.965478082821,-199.660713835502)) ;
#80755=CARTESIAN_POINT('Ctrl Pts',(130.116076731289,-75.915868707821,-199.147382498957)) ;
#80756=CARTESIAN_POINT('Ctrl Pts',(130.842036869422,-75.866259332821,-199.147382498957)) ;
#80757=CARTESIAN_POINT('Ctrl Pts',(131.567997007556,-75.816649957821,-199.147382498957)) ;
#80758=CARTESIAN_POINT('Ctrl Pts',(132.081328344101,-75.767040582821,-199.660713835502)) ;
#80759=CARTESIAN_POINT('Ctrl Pts',(132.594659680647,-75.717431207821,-200.174045172047)) ;
#80760=CARTESIAN_POINT('Ctrl Pts',(132.594659680647,-75.667821832821,-200.900005310181)) ;
#80761=CARTESIAN_POINT('Ctrl Pts',(132.594659680647,-75.618212457821,-201.625965448315)) ;
#80762=CARTESIAN_POINT('Ctrl Pts',(132.081328344101,-75.568603082821,-202.13929678486)) ;
#80763=CARTESIAN_POINT('Ctrl Pts',(131.567997007556,-75.518993707821,-202.652628121405)) ;
#80764=CARTESIAN_POINT('Ctrl Pts',(130.842036869422,-75.469384332821,-202.652628121405)) ;
#80765=CARTESIAN_POINT('Ctrl Pts',(130.116076731289,-75.419774957821,-202.652628121405)) ;
#80766=CARTESIAN_POINT('Ctrl Pts',(129.602745394743,-75.370165582821,-202.13929678486)) ;
#80767=CARTESIAN_POINT('Ctrl Pts',(129.089414058198,-75.320556207821,-201.625965448315)) ;
#80768=CARTESIAN_POINT('Ctrl Pts',(129.089414058198,-75.270946832821,-200.900005310181)) ;
#80769=CARTESIAN_POINT('Ctrl Pts',(129.089414058198,-75.221337457821,-200.174045172048)) ;
#80770=CARTESIAN_POINT('Ctrl Pts',(129.602745394743,-75.171728082821,-199.660713835502)) ;
#80771=CARTESIAN_POINT('Ctrl Pts',(130.116076731289,-75.122118707821,-199.147382498957)) ;
#80772=CARTESIAN_POINT('Ctrl Pts',(130.842036869422,-75.072509332821,-199.147382498957)) ;
#80773=CARTESIAN_POINT('Ctrl Pts',(131.567997007556,-75.022899957821,-199.147382498957)) ;
#80774=CARTESIAN_POINT('Ctrl Pts',(132.081328344101,-74.973290582821,-199.660713835502)) ;
#80775=CARTESIAN_POINT('Ctrl Pts',(132.594659680647,-74.923681207821,-200.174045172047)) ;
#80776=CARTESIAN_POINT('Ctrl Pts',(132.594659680647,-74.874071832821,-200.900005310181)) ;
#80777=CARTESIAN_POINT('Ctrl Pts',(132.594659680647,-74.824462457821,-201.625965448315)) ;
#80778=CARTESIAN_POINT('Ctrl Pts',(132.081328344101,-74.774853082821,-202.13929678486)) ;
#80779=CARTESIAN_POINT('Ctrl Pts',(131.567997007556,-74.725243707821,-202.652628121405)) ;
#80780=CARTESIAN_POINT('Ctrl Pts',(130.842036869422,-74.675634332821,-202.652628121405)) ;
#80781=CARTESIAN_POINT('Ctrl Pts',(130.116076731289,-74.626024957821,-202.652628121405)) ;
#80782=CARTESIAN_POINT('Ctrl Pts',(129.602745394743,-74.576415582821,-202.13929678486)) ;
#80783=CARTESIAN_POINT('Ctrl Pts',(129.089414058198,-74.526806207821,-201.625965448315)) ;
#80784=CARTESIAN_POINT('Ctrl Pts',(129.089414058198,-74.477196832821,-200.900005310181)) ;
#80785=CARTESIAN_POINT('Ctrl Pts',(129.089414058198,-74.427587457821,-200.174045172048)) ;
#80786=CARTESIAN_POINT('Ctrl Pts',(129.602745394743,-74.377978082821,-199.660713835502)) ;
#80787=CARTESIAN_POINT('Ctrl Pts',(130.116076731289,-74.328368707821,-199.147382498957)) ;
#80788=CARTESIAN_POINT('Ctrl Pts',(130.842036869422,-74.278759332821,-199.147382498957)) ;
#80789=CARTESIAN_POINT('Ctrl Pts',(131.567997007556,-74.229149957821,-199.147382498957)) ;
#80790=CARTESIAN_POINT('Ctrl Pts',(132.081328344101,-74.179540582821,-199.660713835502)) ;
#80791=CARTESIAN_POINT('Ctrl Pts',(132.594659680647,-74.129931207821,-200.174045172047)) ;
#80792=CARTESIAN_POINT('Ctrl Pts',(132.594659680647,-74.080321832821,-200.900005310181)) ;
#86293=UNCERTAINTY_MEASURE_WITH_UNIT(LENGTH_MEASURE(0.01),#86331,
'DISTANCE_ACCURACY_VALUE',
'Maximum model space distance between geometric entities at asserted c
onnectivities') ;
#86304=UNCERTAINTY_MEASURE_WITH_UNIT(LENGTH_MEASURE(0.01),#86331,
'DISTANCE_ACCURACY_VALUE',
'Maximum model space distance between geometric entities at asserted c
onnectivities') ;
#86319=(
GEOMETRIC_REPRESENTATION_CONTEXT(3)
GLOBAL_UNCERTAINTY_ASSIGNED_CONTEXT((#86293))
GLOBAL_UNIT_ASSIGNED_CONTEXT((#86331,#86333,#86334))
REPRESENTATION_CONTEXT('','3D')
) ;
#86330=(
GEOMETRIC_REPRESENTATION_CONTEXT(3)
GLOBAL_UNCERTAINTY_ASSIGNED_CONTEXT((#86304))
GLOBAL_UNIT_ASSIGNED_CONTEXT((#86331,#86333,#86334))
REPRESENTATION_CONTEXT('','3D')
) ;
#86331=(
LENGTH_UNIT()
NAMED_UNIT(*)
SI_UNIT(.MILLI.,.METRE.)
) ;
#86333=(
NAMED_UNIT(*)
PLANE_ANGLE_UNIT()
SI_UNIT($,.RADIAN.)
) ;
#86334=(
NAMED_UNIT(*)
SI_UNIT($,.STERADIAN.)
SOLID_ANGLE_UNIT()
) ;
#86349=SHAPE_DEFINITION_REPRESENTATION(#86398,#86465) ;
#86398=PRODUCT_DEFINITION_SHAPE('',$,#86491) ;
#86465=SHAPE_REPRESENTATION('',(#35912),#86319) ;
#86476=PRODUCT_DEFINITION_CONTEXT('part definition',#86553,'design') ;
#86491=PRODUCT_DEFINITION('Squash_Plate','Squash_Plate',#86516,#86476) ;
#86516=PRODUCT_DEFINITION_FORMATION('',$,#86569) ;
#86553=APPLICATION_CONTEXT(
'Core Data for Automotive Mechanical Design Process') ;
#86554=PRODUCT_CONTEXT('part definition',#86553,'mechanical') ;
#86569=PRODUCT('Squash_Plate','Squash_Plate',$,(#86554)) ;
#86582=PRESENTATION_STYLE_ASSIGNMENT((#86587)) ;
#86587=SURFACE_STYLE_USAGE(.BOTH.,#86592) ;
#86592=SURFACE_SIDE_STYLE('',(#86597)) ;
#86597=SURFACE_STYLE_FILL_AREA(#86602) ;
#86602=FILL_AREA_STYLE('Opaque(203,203,203)',(#86607)) ;
#86607=FILL_AREA_STYLE_COLOUR('Opaque(203,203,203)',#86612) ;
#86612=COLOUR_RGB('Opaque(203,203,203)', 0.66274510, 0.83137255, 0.94901961) ;
ENDSEC;
END-ISO-10303-21;
